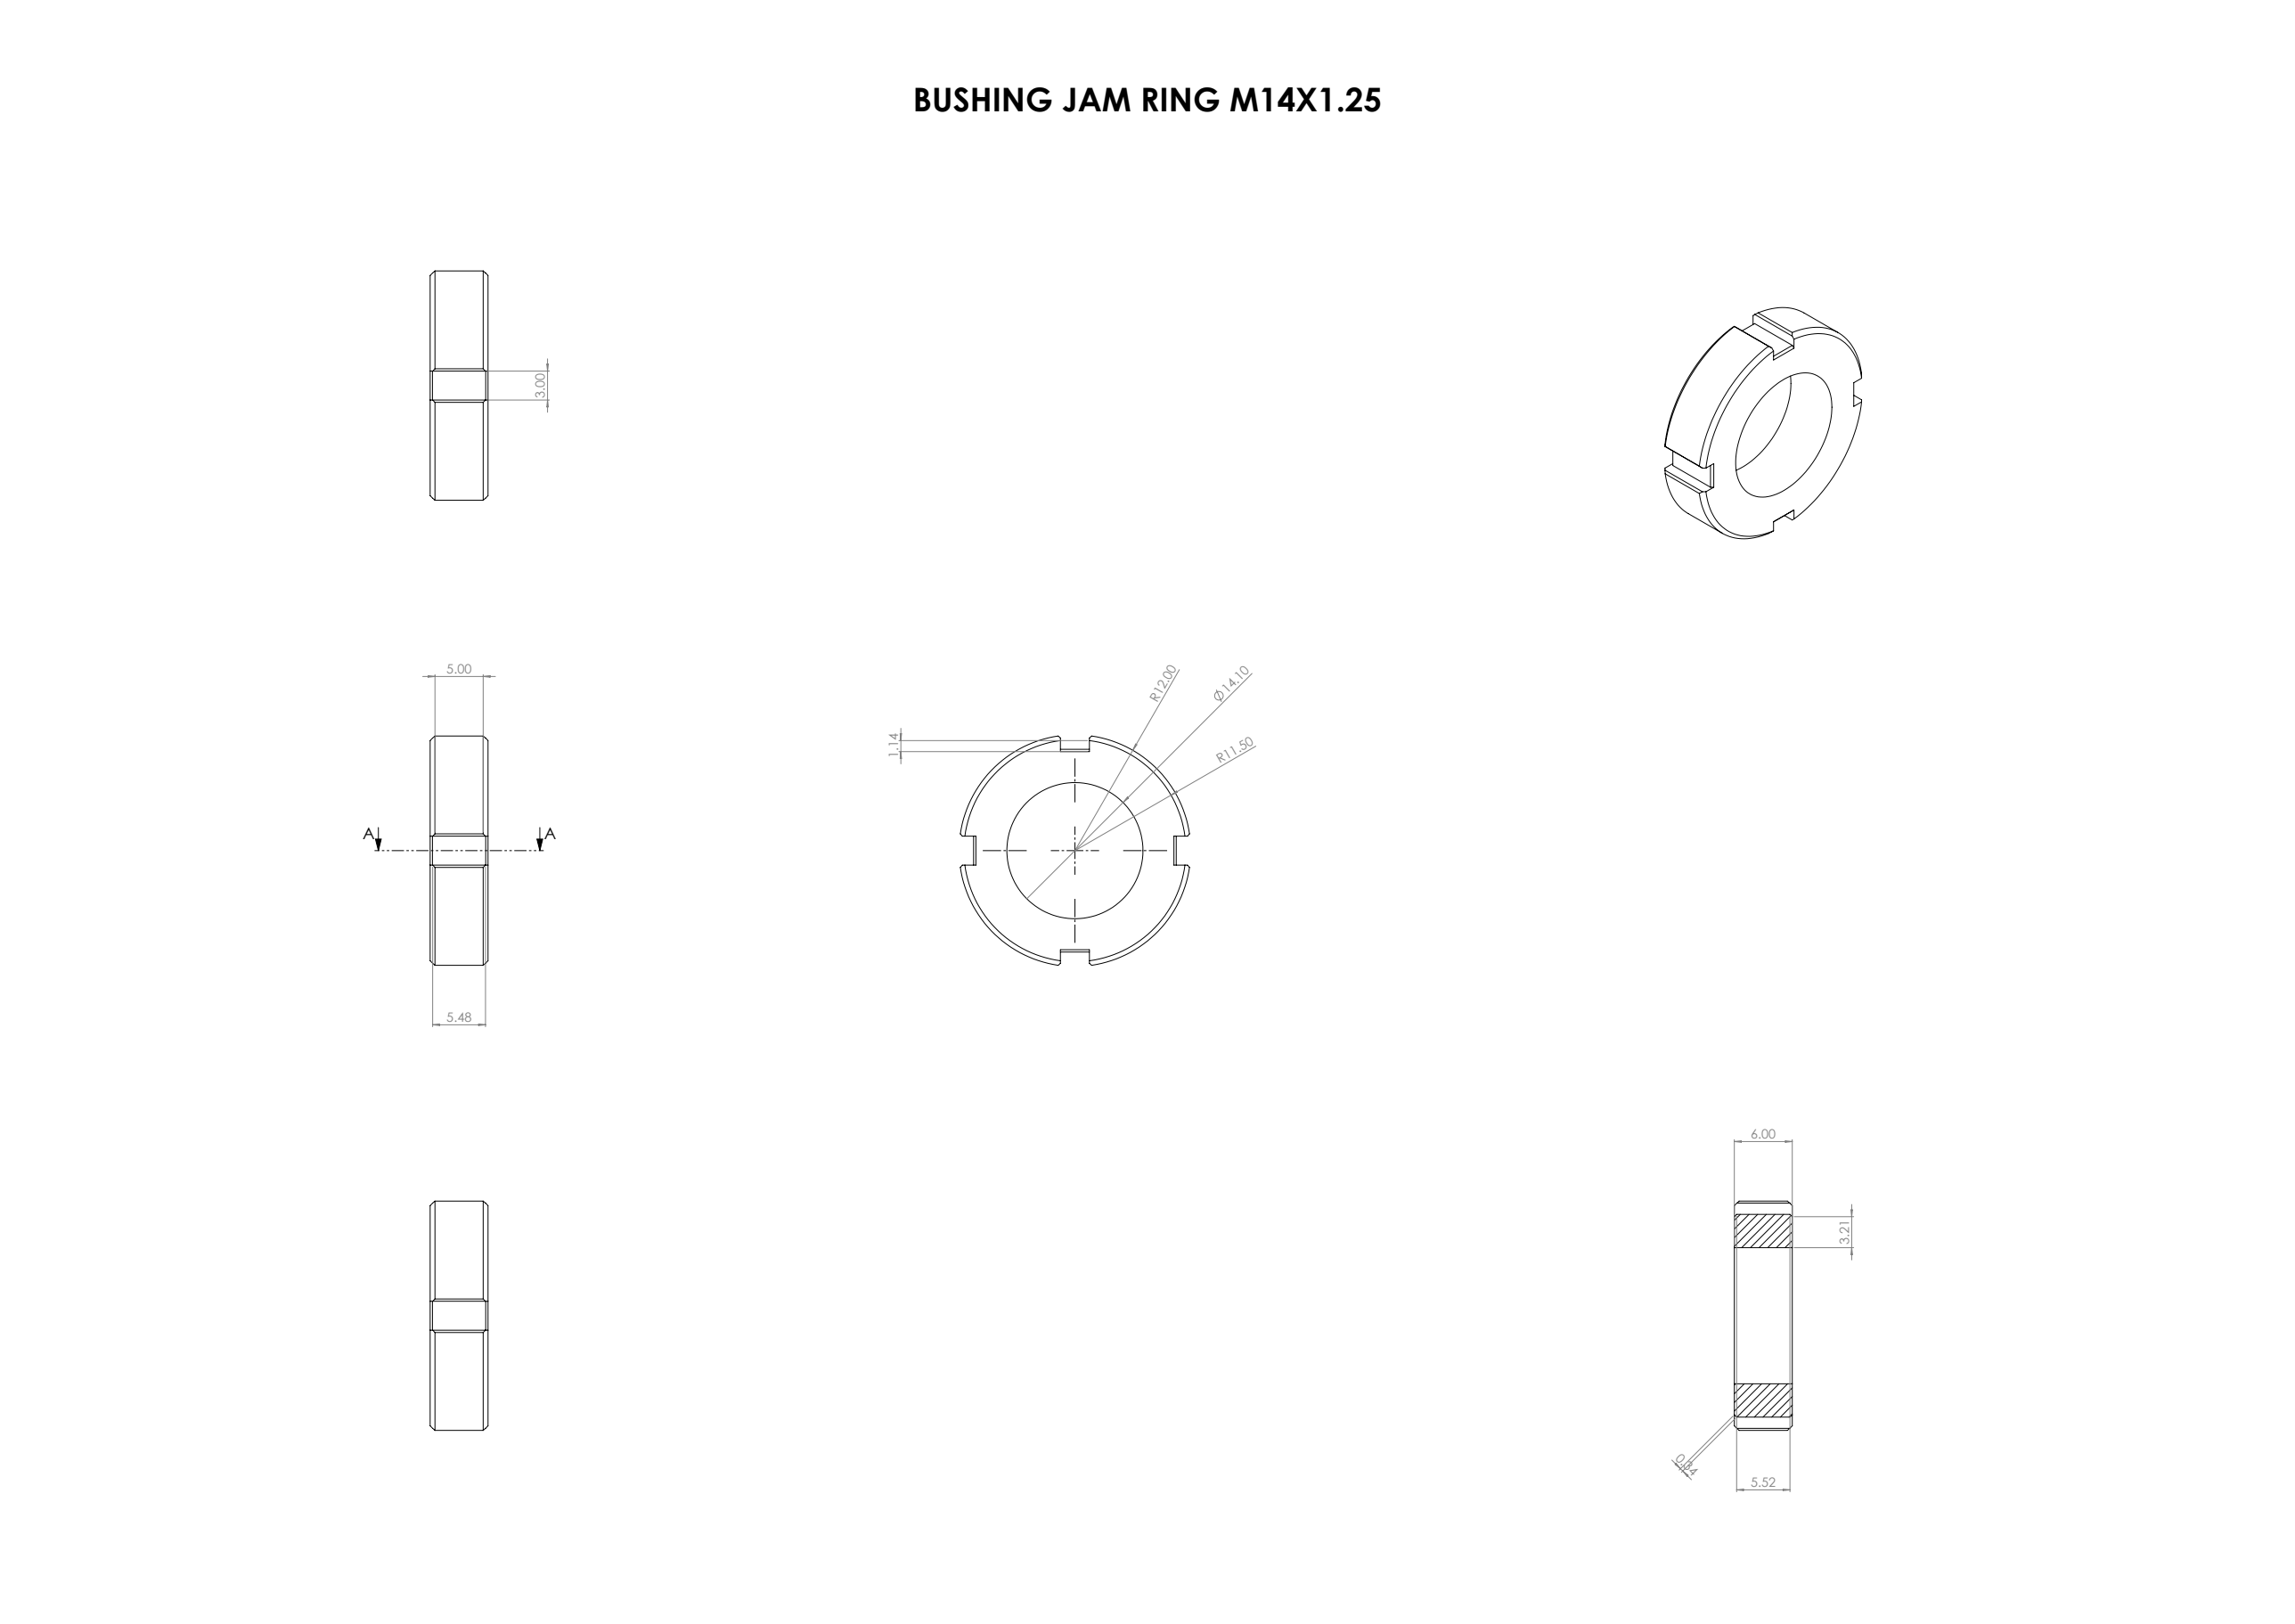
ISO-10303-21;
HEADER;
/* Generated by software containing ST-Developer
 * from STEP Tools, Inc. (www.steptools.com) 
 */

FILE_DESCRIPTION(
/* description */ (''),
/* implementation_level */ '2;1');

FILE_NAME(
/* name */ '08_Bushing_Jam_Ring_M14x1.25.step',
/* time_stamp */ '2026-10-21T01:56:51-07:00',
/* author */ (''),
/* organization */ (''),
/* preprocessor_version */ 'ST-DEVELOPER v20.2',
/* originating_system */ 'Autodesk Translation Framework v15.15.0.0',
/* authorisation */ '');

FILE_SCHEMA (('AUTOMOTIVE_DESIGN { 1 0 10303 214 3 1 1 }'));
ENDSEC;

DATA;
#10=MECHANICAL_DESIGN_GEOMETRIC_PRESENTATION_REPRESENTATION('',(#284),#82384);
#170=(
BOUNDED_CURVE()
B_SPLINE_CURVE(2,(#65757,#65758,#65759),.UNSPECIFIED.,.F.,.F.)
B_SPLINE_CURVE_WITH_KNOTS((3,3),(0.0445378083500862,0.0835095062261198),
 .UNSPECIFIED.)
CURVE()
GEOMETRIC_REPRESENTATION_ITEM()
RATIONAL_B_SPLINE_CURVE((1.00020174547405,1.00018913890855,1.))
REPRESENTATION_ITEM('')
);
#171=(
BOUNDED_CURVE()
B_SPLINE_CURVE(2,(#65763,#65764,#65765),.UNSPECIFIED.,.F.,.F.)
B_SPLINE_CURVE_WITH_KNOTS((3,3),(0.,0.0389716978752448),.UNSPECIFIED.)
CURVE()
GEOMETRIC_REPRESENTATION_ITEM()
RATIONAL_B_SPLINE_CURVE((1.,1.0001891389102,1.00020174547581))
REPRESENTATION_ITEM('')
);
#172=(
BOUNDED_CURVE()
B_SPLINE_CURVE(2,(#65775,#65776,#65777),.UNSPECIFIED.,.F.,.F.)
B_SPLINE_CURVE_WITH_KNOTS((3,3),(0.033425828127436,0.0710030761269733),
 .UNSPECIFIED.)
CURVE()
GEOMETRIC_REPRESENTATION_ITEM()
RATIONAL_B_SPLINE_CURVE((1.0001146955549,1.00012181803223,1.))
REPRESENTATION_ITEM('')
);
#173=(
BOUNDED_CURVE()
B_SPLINE_CURVE(2,(#65781,#65782,#65783),.UNSPECIFIED.,.F.,.F.)
B_SPLINE_CURVE_WITH_KNOTS((3,3),(0.,0.0375772479994726),.UNSPECIFIED.)
CURVE()
GEOMETRIC_REPRESENTATION_ITEM()
RATIONAL_B_SPLINE_CURVE((1.,1.00012181795416,1.0001146954814))
REPRESENTATION_ITEM('')
);
#174=(
BOUNDED_CURVE()
B_SPLINE_CURVE(2,(#65784,#65785,#65786),.UNSPECIFIED.,.F.,.F.)
B_SPLINE_CURVE_WITH_KNOTS((3,3),(0.,0.0389716978752398),.UNSPECIFIED.)
CURVE()
GEOMETRIC_REPRESENTATION_ITEM()
RATIONAL_B_SPLINE_CURVE((1.,1.00018913890916,1.0002017454747))
REPRESENTATION_ITEM('')
);
#175=(
BOUNDED_CURVE()
B_SPLINE_CURVE(2,(#65790,#65791,#65792),.UNSPECIFIED.,.F.,.F.)
B_SPLINE_CURVE_WITH_KNOTS((3,3),(0.0445378083500902,0.0835095062261194),
 .UNSPECIFIED.)
CURVE()
GEOMETRIC_REPRESENTATION_ITEM()
RATIONAL_B_SPLINE_CURVE((1.00020174547445,1.00018913890892,1.))
REPRESENTATION_ITEM('')
);
#176=(
BOUNDED_CURVE()
B_SPLINE_CURVE(2,(#65796,#65797,#65798),.UNSPECIFIED.,.F.,.F.)
B_SPLINE_CURVE_WITH_KNOTS((3,3),(0.,0.0389716978752542),.UNSPECIFIED.)
CURVE()
GEOMETRIC_REPRESENTATION_ITEM()
RATIONAL_B_SPLINE_CURVE((1.,1.00018913890855,1.00020174547405))
REPRESENTATION_ITEM('')
);
#177=(
BOUNDED_CURVE()
B_SPLINE_CURVE(2,(#65802,#65803,#65804),.UNSPECIFIED.,.F.,.F.)
B_SPLINE_CURVE_WITH_KNOTS((3,3),(0.,0.0375772479995372),.UNSPECIFIED.)
CURVE()
GEOMETRIC_REPRESENTATION_ITEM()
RATIONAL_B_SPLINE_CURVE((1.,1.00012181803223,1.0001146955549))
REPRESENTATION_ITEM('')
);
#178=(
BOUNDED_CURVE()
B_SPLINE_CURVE(2,(#65810,#65811,#65812),.UNSPECIFIED.,.F.,.F.)
B_SPLINE_CURVE_WITH_KNOTS((3,3),(0.0334258281258571,0.0710030761269732),
 .UNSPECIFIED.)
CURVE()
GEOMETRIC_REPRESENTATION_ITEM()
RATIONAL_B_SPLINE_CURVE((1.00011469550903,1.00012181798351,1.))
REPRESENTATION_ITEM('')
);
#179=(
BOUNDED_CURVE()
B_SPLINE_CURVE(2,(#65817,#65818,#65819),.UNSPECIFIED.,.F.,.F.)
B_SPLINE_CURVE_WITH_KNOTS((3,3),(0.044537808350094,0.0835095062261198),
 .UNSPECIFIED.)
CURVE()
GEOMETRIC_REPRESENTATION_ITEM()
RATIONAL_B_SPLINE_CURVE((1.00020174547469,1.00018913890915,1.))
REPRESENTATION_ITEM('')
);
#180=(
BOUNDED_CURVE()
B_SPLINE_CURVE(2,(#65821,#65822,#65823),.UNSPECIFIED.,.F.,.F.)
B_SPLINE_CURVE_WITH_KNOTS((3,3),(0.0334258281275199,0.0710030761269733),
 .UNSPECIFIED.)
CURVE()
GEOMETRIC_REPRESENTATION_ITEM()
RATIONAL_B_SPLINE_CURVE((1.00011469547359,1.00012181794587,1.))
REPRESENTATION_ITEM('')
);
#181=(
BOUNDED_CURVE()
B_SPLINE_CURVE(2,(#65844,#65845,#65846),.UNSPECIFIED.,.F.,.F.)
B_SPLINE_CURVE_WITH_KNOTS((3,3),(0.,0.0389716978752325),.UNSPECIFIED.)
CURVE()
GEOMETRIC_REPRESENTATION_ITEM()
RATIONAL_B_SPLINE_CURVE((1.,1.00018913890989,1.00020174547548))
REPRESENTATION_ITEM('')
);
#182=(
BOUNDED_CURVE()
B_SPLINE_CURVE(2,(#65850,#65851,#65852),.UNSPECIFIED.,.F.,.F.)
B_SPLINE_CURVE_WITH_KNOTS((3,3),(0.,0.0375772480011104),.UNSPECIFIED.)
CURVE()
GEOMETRIC_REPRESENTATION_ITEM()
RATIONAL_B_SPLINE_CURVE((1.,1.00012181798092,1.00011469550659))
REPRESENTATION_ITEM('')
);
#183=(
BOUNDED_CURVE()
B_SPLINE_CURVE(2,(#65860,#65861,#65862),.UNSPECIFIED.,.F.,.F.)
B_SPLINE_CURVE_WITH_KNOTS((3,3),(0.0445378083500976,0.0835095062261196),
 .UNSPECIFIED.)
CURVE()
GEOMETRIC_REPRESENTATION_ITEM()
RATIONAL_B_SPLINE_CURVE((1.0002017454746,1.00018913890906,1.))
REPRESENTATION_ITEM('')
);
#184=(
BOUNDED_CURVE()
B_SPLINE_CURVE(2,(#65866,#65867,#65868),.UNSPECIFIED.,.F.,.F.)
B_SPLINE_CURVE_WITH_KNOTS((3,3),(0.,0.0389716978752574),.UNSPECIFIED.)
CURVE()
GEOMETRIC_REPRESENTATION_ITEM()
RATIONAL_B_SPLINE_CURVE((1.,1.00018913890786,1.00020174547332))
REPRESENTATION_ITEM('')
);
#185=(
BOUNDED_CURVE()
B_SPLINE_CURVE(2,(#65878,#65879,#65880),.UNSPECIFIED.,.F.,.F.)
B_SPLINE_CURVE_WITH_KNOTS((3,3),(0.0334258281258531,0.0710030761269732),
 .UNSPECIFIED.)
CURVE()
GEOMETRIC_REPRESENTATION_ITEM()
RATIONAL_B_SPLINE_CURVE((1.00011469551065,1.00012181798524,1.))
REPRESENTATION_ITEM('')
);
#186=(
BOUNDED_CURVE()
B_SPLINE_CURVE(2,(#65884,#65885,#65886),.UNSPECIFIED.,.F.,.F.)
B_SPLINE_CURVE_WITH_KNOTS((3,3),(0.,0.0375772480011044),.UNSPECIFIED.)
CURVE()
GEOMETRIC_REPRESENTATION_ITEM()
RATIONAL_B_SPLINE_CURVE((1.,1.00012181797833,1.00011469550415))
REPRESENTATION_ITEM('')
);
#187=(
BOUNDED_CURVE()
B_SPLINE_CURVE(2,(#65887,#65888,#65889),.UNSPECIFIED.,.F.,.F.)
B_SPLINE_CURVE_WITH_KNOTS((3,3),(0.,0.0389716978752387),.UNSPECIFIED.)
CURVE()
GEOMETRIC_REPRESENTATION_ITEM()
RATIONAL_B_SPLINE_CURVE((1.,1.00018913890938,1.00020174547494))
REPRESENTATION_ITEM('')
);
#188=(
BOUNDED_CURVE()
B_SPLINE_CURVE(2,(#65907,#65908,#65909),.UNSPECIFIED.,.F.,.F.)
B_SPLINE_CURVE_WITH_KNOTS((3,3),(0.0445378083500854,0.0835095062261198),
 .UNSPECIFIED.)
CURVE()
GEOMETRIC_REPRESENTATION_ITEM()
RATIONAL_B_SPLINE_CURVE((1.00020174547577,1.00018913891016,1.))
REPRESENTATION_ITEM('')
);
#189=(
BOUNDED_CURVE()
B_SPLINE_CURVE(2,(#65913,#65914,#65915),.UNSPECIFIED.,.F.,.F.)
B_SPLINE_CURVE_WITH_KNOTS((3,3),(0.0334258281275259,0.0710030761269733),
 .UNSPECIFIED.)
CURVE()
GEOMETRIC_REPRESENTATION_ITEM()
RATIONAL_B_SPLINE_CURVE((1.00011469547113,1.00012181794325,1.))
REPRESENTATION_ITEM('')
);
#190=(
BOUNDED_CURVE()
B_SPLINE_CURVE(2,(#65918,#65919,#65920),.UNSPECIFIED.,.F.,.F.)
B_SPLINE_CURVE_WITH_KNOTS((3,3),(0.,0.0375772479994632),.UNSPECIFIED.)
CURVE()
GEOMETRIC_REPRESENTATION_ITEM()
RATIONAL_B_SPLINE_CURVE((1.,1.00012181795023,1.0001146954777))
REPRESENTATION_ITEM('')
);
#191=(
BOUNDED_CURVE()
B_SPLINE_CURVE(2,(#65929,#65930,#65931),.UNSPECIFIED.,.F.,.F.)
B_SPLINE_CURVE_WITH_KNOTS((3,3),(0.044537808350101,0.0835095062261195),
 .UNSPECIFIED.)
CURVE()
GEOMETRIC_REPRESENTATION_ITEM()
RATIONAL_B_SPLINE_CURVE((1.00020174547522,1.00018913890965,1.))
REPRESENTATION_ITEM('')
);
#192=(
BOUNDED_CURVE()
B_SPLINE_CURVE(2,(#65935,#65936,#65937),.UNSPECIFIED.,.F.,.F.)
B_SPLINE_CURVE_WITH_KNOTS((3,3),(0.,0.0389716978752438),.UNSPECIFIED.)
CURVE()
GEOMETRIC_REPRESENTATION_ITEM()
RATIONAL_B_SPLINE_CURVE((1.,1.00018913890923,1.00020174547478))
REPRESENTATION_ITEM('')
);
#193=(
BOUNDED_CURVE()
B_SPLINE_CURVE(2,(#65947,#65948,#65949),.UNSPECIFIED.,.F.,.F.)
B_SPLINE_CURVE_WITH_KNOTS((3,3),(0.0334258281258831,0.0710030761269732),
 .UNSPECIFIED.)
CURVE()
GEOMETRIC_REPRESENTATION_ITEM()
RATIONAL_B_SPLINE_CURVE((1.00011469550092,1.0001218179749,1.))
REPRESENTATION_ITEM('')
);
#194=(
BOUNDED_CURVE()
B_SPLINE_CURVE(2,(#65953,#65954,#65955),.UNSPECIFIED.,.F.,.F.)
B_SPLINE_CURVE_WITH_KNOTS((3,3),(0.,0.0375772480008883),.UNSPECIFIED.)
CURVE()
GEOMETRIC_REPRESENTATION_ITEM()
RATIONAL_B_SPLINE_CURVE((1.,1.0001218179815,1.00011469550713))
REPRESENTATION_ITEM('')
);
#195=(
BOUNDED_CURVE()
B_SPLINE_CURVE(2,(#65956,#65957,#65958),.UNSPECIFIED.,.F.,.F.)
B_SPLINE_CURVE_WITH_KNOTS((3,3),(0.,0.0389716978752413),.UNSPECIFIED.)
CURVE()
GEOMETRIC_REPRESENTATION_ITEM()
RATIONAL_B_SPLINE_CURVE((1.,1.00018913890951,1.00020174547507))
REPRESENTATION_ITEM('')
);
#196=(
BOUNDED_CURVE()
B_SPLINE_CURVE(2,(#65994,#65995,#65996),.UNSPECIFIED.,.F.,.F.)
B_SPLINE_CURVE_WITH_KNOTS((3,3),(0.0445378083501022,0.0835095062261196),
 .UNSPECIFIED.)
CURVE()
GEOMETRIC_REPRESENTATION_ITEM()
RATIONAL_B_SPLINE_CURVE((1.00020174547498,1.00018913890943,1.))
REPRESENTATION_ITEM('')
);
#197=(
BOUNDED_CURVE()
B_SPLINE_CURVE(2,(#66000,#66001,#66002),.UNSPECIFIED.,.F.,.F.)
B_SPLINE_CURVE_WITH_KNOTS((3,3),(0.0334258281258389,0.0710030761269732),
 .UNSPECIFIED.)
CURVE()
GEOMETRIC_REPRESENTATION_ITEM()
RATIONAL_B_SPLINE_CURVE((1.00011469551635,1.00012181799128,1.))
REPRESENTATION_ITEM('')
);
#198=(
BOUNDED_CURVE()
B_SPLINE_CURVE(2,(#66005,#66006,#66007),.UNSPECIFIED.,.F.,.F.)
B_SPLINE_CURVE_WITH_KNOTS((3,3),(0.,0.0375772480011161),.UNSPECIFIED.)
CURVE()
GEOMETRIC_REPRESENTATION_ITEM()
RATIONAL_B_SPLINE_CURVE((1.,1.00012181798351,1.00011469550903))
REPRESENTATION_ITEM('')
);
#199=(
BOUNDED_CURVE()
B_SPLINE_CURVE(2,(#66013,#66014,#66015),.UNSPECIFIED.,.F.,.F.)
B_SPLINE_CURVE_WITH_KNOTS((3,3),(0.0445378083500857,0.0835095062261197),
 .UNSPECIFIED.)
CURVE()
GEOMETRIC_REPRESENTATION_ITEM()
RATIONAL_B_SPLINE_CURVE((1.00020174547356,1.0001891389081,1.))
REPRESENTATION_ITEM('')
);
#200=(
BOUNDED_CURVE()
B_SPLINE_CURVE(2,(#66019,#66020,#66021),.UNSPECIFIED.,.F.,.F.)
B_SPLINE_CURVE_WITH_KNOTS((3,3),(0.03342582812753,0.0710030761269734),
 .UNSPECIFIED.)
CURVE()
GEOMETRIC_REPRESENTATION_ITEM()
RATIONAL_B_SPLINE_CURVE((1.00011469546948,1.0001218179415,1.))
REPRESENTATION_ITEM('')
);
#201=(
BOUNDED_CURVE()
B_SPLINE_CURVE(2,(#66024,#66025,#66026),.UNSPECIFIED.,.F.,.F.)
B_SPLINE_CURVE_WITH_KNOTS((3,3),(0.,0.0375772479994669),.UNSPECIFIED.)
CURVE()
GEOMETRIC_REPRESENTATION_ITEM()
RATIONAL_B_SPLINE_CURVE((1.,1.00012181795155,1.00011469547894))
REPRESENTATION_ITEM('')
);
#246=SHAPE_REPRESENTATION_RELATIONSHIP('SRR','None',#82480,#265);
#265=ADVANCED_BREP_SHAPE_REPRESENTATION('',(#303),#82379);
#284=STYLED_ITEM('',(#82645),#303);
#303=MANIFOLD_SOLID_BREP('Body1',#30675);
#807=CYLINDRICAL_SURFACE('',#32849,12.);
#808=CYLINDRICAL_SURFACE('',#32864,12.);
#809=CYLINDRICAL_SURFACE('',#32876,12.);
#810=CYLINDRICAL_SURFACE('',#32900,12.);
#811=CYLINDRICAL_SURFACE('',#32904,7.05);
#1724=CIRCLE('',#32850,12.);
#1725=CIRCLE('',#32851,12.);
#1726=CIRCLE('',#32853,11.5);
#1727=CIRCLE('',#32857,12.);
#1728=CIRCLE('',#32858,11.5);
#1729=CIRCLE('',#32865,12.);
#1730=CIRCLE('',#32866,12.);
#1731=CIRCLE('',#32868,11.5);
#1732=CIRCLE('',#32873,11.5);
#1733=CIRCLE('',#32877,12.);
#1734=CIRCLE('',#32878,12.);
#1735=CIRCLE('',#32880,11.5);
#1736=CIRCLE('',#32889,11.5);
#1737=CIRCLE('',#32893,11.5);
#1738=CIRCLE('',#32896,11.5);
#1739=CIRCLE('',#32897,7.05);
#1740=CIRCLE('',#32901,12.);
#1741=CIRCLE('',#32905,7.05);
#2047=CONICAL_SURFACE('',#32852,11.75,0.78539816339745);
#2048=CONICAL_SURFACE('',#32856,11.75,0.78539816339745);
#2049=CONICAL_SURFACE('',#32867,11.75,0.785398163397449);
#2050=CONICAL_SURFACE('',#32872,11.75,0.78539816339745);
#2051=CONICAL_SURFACE('',#32879,11.75,0.785398163397449);
#2052=CONICAL_SURFACE('',#32888,11.75,0.785398163397449);
#2053=CONICAL_SURFACE('',#32892,11.75,0.78539816339745);
#2054=CONICAL_SURFACE('',#32902,11.75,0.785398163397449);
#3564=FACE_BOUND('',#7019,.T.);
#3565=FACE_BOUND('',#7027,.T.);
#4947=FACE_OUTER_BOUND('',#6983,.T.);
#4948=FACE_OUTER_BOUND('',#6984,.T.);
#4949=FACE_OUTER_BOUND('',#6985,.T.);
#4950=FACE_OUTER_BOUND('',#6986,.T.);
#4951=FACE_OUTER_BOUND('',#6987,.T.);
#4952=FACE_OUTER_BOUND('',#6988,.T.);
#4953=FACE_OUTER_BOUND('',#6989,.T.);
#4954=FACE_OUTER_BOUND('',#6990,.T.);
#4955=FACE_OUTER_BOUND('',#6991,.T.);
#4956=FACE_OUTER_BOUND('',#6992,.T.);
#4957=FACE_OUTER_BOUND('',#6993,.T.);
#4958=FACE_OUTER_BOUND('',#6994,.T.);
#4959=FACE_OUTER_BOUND('',#6995,.T.);
#4960=FACE_OUTER_BOUND('',#6996,.T.);
#4961=FACE_OUTER_BOUND('',#6997,.T.);
#4962=FACE_OUTER_BOUND('',#6998,.T.);
#4963=FACE_OUTER_BOUND('',#6999,.T.);
#4964=FACE_OUTER_BOUND('',#7000,.T.);
#4965=FACE_OUTER_BOUND('',#7001,.T.);
#4966=FACE_OUTER_BOUND('',#7002,.T.);
#4967=FACE_OUTER_BOUND('',#7003,.T.);
#4968=FACE_OUTER_BOUND('',#7004,.T.);
#4969=FACE_OUTER_BOUND('',#7005,.T.);
#4970=FACE_OUTER_BOUND('',#7006,.T.);
#4971=FACE_OUTER_BOUND('',#7007,.T.);
#4972=FACE_OUTER_BOUND('',#7008,.T.);
#4973=FACE_OUTER_BOUND('',#7009,.T.);
#4974=FACE_OUTER_BOUND('',#7010,.T.);
#4975=FACE_OUTER_BOUND('',#7011,.T.);
#4976=FACE_OUTER_BOUND('',#7012,.T.);
#4977=FACE_OUTER_BOUND('',#7013,.T.);
#4978=FACE_OUTER_BOUND('',#7014,.T.);
#4979=FACE_OUTER_BOUND('',#7015,.T.);
#4980=FACE_OUTER_BOUND('',#7016,.T.);
#4981=FACE_OUTER_BOUND('',#7017,.T.);
#4982=FACE_OUTER_BOUND('',#7018,.T.);
#4983=FACE_OUTER_BOUND('',#7020,.T.);
#4984=FACE_OUTER_BOUND('',#7021,.T.);
#4985=FACE_OUTER_BOUND('',#7022,.T.);
#4986=FACE_OUTER_BOUND('',#7023,.T.);
#4987=FACE_OUTER_BOUND('',#7024,.T.);
#4988=FACE_OUTER_BOUND('',#7025,.T.);
#4989=FACE_OUTER_BOUND('',#7026,.T.);
#6983=EDGE_LOOP('',(#25917,#25918,#25919,#25920));
#6984=EDGE_LOOP('',(#25921,#25922,#25923,#25924));
#6985=EDGE_LOOP('',(#25925,#25926,#25927,#25928));
#6986=EDGE_LOOP('',(#25929,#25930,#25931,#25932));
#6987=EDGE_LOOP('',(#25933,#25934,#25935,#25936,#25937,#25938));
#6988=EDGE_LOOP('',(#25939,#25940,#25941,#25942));
#6989=EDGE_LOOP('',(#25943,#25944,#25945,#25946,#25947,#25948,#25949,#25950));
#6990=EDGE_LOOP('',(#25951,#25952,#25953,#25954,#25955,#25956));
#6991=EDGE_LOOP('',(#25957,#25958,#25959,#25960));
#6992=EDGE_LOOP('',(#25961,#25962,#25963,#25964));
#6993=EDGE_LOOP('',(#25965,#25966,#25967,#25968));
#6994=EDGE_LOOP('',(#25969,#25970,#25971,#25972,#25973,#25974,#25975,#25976));
#6995=EDGE_LOOP('',(#25977,#25978,#25979,#25980));
#6996=EDGE_LOOP('',(#25981,#25982,#25983,#25984));
#6997=EDGE_LOOP('',(#25985,#25986,#25987,#25988,#25989,#25990));
#6998=EDGE_LOOP('',(#25991,#25992,#25993,#25994));
#6999=EDGE_LOOP('',(#25995,#25996,#25997,#25998));
#7000=EDGE_LOOP('',(#25999,#26000,#26001,#26002));
#7001=EDGE_LOOP('',(#26003,#26004,#26005,#26006,#26007,#26008));
#7002=EDGE_LOOP('',(#26009,#26010,#26011,#26012,#26013,#26014,#26015,#26016));
#7003=EDGE_LOOP('',(#26017,#26018,#26019,#26020));
#7004=EDGE_LOOP('',(#26021,#26022,#26023,#26024));
#7005=EDGE_LOOP('',(#26025,#26026,#26027,#26028,#26029,#26030));
#7006=EDGE_LOOP('',(#26031,#26032,#26033,#26034));
#7007=EDGE_LOOP('',(#26035,#26036,#26037,#26038));
#7008=EDGE_LOOP('',(#26039,#26040,#26041,#26042));
#7009=EDGE_LOOP('',(#26043,#26044,#26045,#26046));
#7010=EDGE_LOOP('',(#26047,#26048,#26049,#26050));
#7011=EDGE_LOOP('',(#26051,#26052,#26053,#26054));
#7012=EDGE_LOOP('',(#26055,#26056,#26057,#26058));
#7013=EDGE_LOOP('',(#26059,#26060,#26061,#26062,#26063,#26064));
#7014=EDGE_LOOP('',(#26065,#26066,#26067,#26068,#26069,#26070,#26071,#26072));
#7015=EDGE_LOOP('',(#26073,#26074,#26075,#26076));
#7016=EDGE_LOOP('',(#26077,#26078,#26079,#26080,#26081,#26082));
#7017=EDGE_LOOP('',(#26083,#26084,#26085,#26086,#26087,#26088,#26089,#26090));
#7018=EDGE_LOOP('',(#26091,#26092,#26093,#26094,#26095,#26096,#26097,#26098,
#26099,#26100,#26101,#26102,#26103,#26104,#26105,#26106));
#7019=EDGE_LOOP('',(#26107));
#7020=EDGE_LOOP('',(#26108,#26109,#26110,#26111,#26112,#26113,#26114,#26115));
#7021=EDGE_LOOP('',(#26116,#26117,#26118,#26119,#26120,#26121,#26122,#26123));
#7022=EDGE_LOOP('',(#26124,#26125,#26126,#26127));
#7023=EDGE_LOOP('',(#26128,#26129,#26130,#26131,#26132,#26133));
#7024=EDGE_LOOP('',(#26134,#26135,#26136,#26137,#26138,#26139,#26140,#26141));
#7025=EDGE_LOOP('',(#26142,#26143,#26144,#26145));
#7026=EDGE_LOOP('',(#26146,#26147,#26148,#26149,#26150,#26151,#26152,#26153,
#26154,#26155,#26156,#26157,#26158,#26159,#26160,#26161));
#7027=EDGE_LOOP('',(#26162));
#9258=LINE('',#65742,#11564);
#9259=LINE('',#65744,#11565);
#9260=LINE('',#65746,#11566);
#9261=LINE('',#65747,#11567);
#9262=LINE('',#65750,#11568);
#9263=LINE('',#65752,#11569);
#9264=LINE('',#65753,#11570);
#9265=LINE('',#65761,#11571);
#9266=LINE('',#65766,#11572);
#9267=LINE('',#65771,#11573);
#9268=LINE('',#65794,#11574);
#9269=LINE('',#65799,#11575);
#9270=LINE('',#65805,#11576);
#9271=LINE('',#65807,#11577);
#9272=LINE('',#65809,#11578);
#9273=LINE('',#65828,#11579);
#9274=LINE('',#65830,#11580);
#9275=LINE('',#65832,#11581);
#9276=LINE('',#65833,#11582);
#9277=LINE('',#65836,#11583);
#9278=LINE('',#65838,#11584);
#9279=LINE('',#65839,#11585);
#9280=LINE('',#65842,#11586);
#9281=LINE('',#65847,#11587);
#9282=LINE('',#65854,#11588);
#9283=LINE('',#65855,#11589);
#9284=LINE('',#65856,#11590);
#9285=LINE('',#65864,#11591);
#9286=LINE('',#65869,#11592);
#9287=LINE('',#65874,#11593);
#9288=LINE('',#65893,#11594);
#9289=LINE('',#65895,#11595);
#9290=LINE('',#65897,#11596);
#9291=LINE('',#65898,#11597);
#9292=LINE('',#65901,#11598);
#9293=LINE('',#65903,#11599);
#9294=LINE('',#65904,#11600);
#9295=LINE('',#65910,#11601);
#9296=LINE('',#65923,#11602);
#9297=LINE('',#65924,#11603);
#9298=LINE('',#65925,#11604);
#9299=LINE('',#65933,#11605);
#9300=LINE('',#65938,#11606);
#9301=LINE('',#65943,#11607);
#9302=LINE('',#65961,#11608);
#9303=LINE('',#65962,#11609);
#9304=LINE('',#65965,#11610);
#9305=LINE('',#65966,#11611);
#9306=LINE('',#65969,#11612);
#9307=LINE('',#65970,#11613);
#9308=LINE('',#65974,#11614);
#9309=LINE('',#65976,#11615);
#9310=LINE('',#65978,#11616);
#9311=LINE('',#65979,#11617);
#9312=LINE('',#65982,#11618);
#9313=LINE('',#65984,#11619);
#9314=LINE('',#65985,#11620);
#9315=LINE('',#65988,#11621);
#9316=LINE('',#65990,#11622);
#9317=LINE('',#65991,#11623);
#9318=LINE('',#65997,#11624);
#9319=LINE('',#66009,#11625);
#9320=LINE('',#66010,#11626);
#9321=LINE('',#66016,#11627);
#9322=LINE('',#66028,#11628);
#9323=LINE('',#66029,#11629);
#9324=LINE('',#66031,#11630);
#9325=LINE('',#66032,#11631);
#9326=LINE('',#66033,#11632);
#9327=LINE('',#66038,#11633);
#9328=LINE('',#66040,#11634);
#9329=LINE('',#66045,#11635);
#9330=LINE('',#66049,#11636);
#11564=VECTOR('',#39203,10.);
#11565=VECTOR('',#39204,10.);
#11566=VECTOR('',#39205,10.);
#11567=VECTOR('',#39206,10.);
#11568=VECTOR('',#39209,10.);
#11569=VECTOR('',#39210,10.);
#11570=VECTOR('',#39211,10.);
#11571=VECTOR('',#39214,10.);
#11572=VECTOR('',#39215,10.);
#11573=VECTOR('',#39220,10.);
#11574=VECTOR('',#39229,10.);
#11575=VECTOR('',#39230,10.);
#11576=VECTOR('',#39233,10.);
#11577=VECTOR('',#39234,10.);
#11578=VECTOR('',#39235,10.);
#11579=VECTOR('',#39244,10.);
#11580=VECTOR('',#39245,10.);
#11581=VECTOR('',#39246,10.);
#11582=VECTOR('',#39247,10.);
#11583=VECTOR('',#39250,10.);
#11584=VECTOR('',#39251,10.);
#11585=VECTOR('',#39252,10.);
#11586=VECTOR('',#39255,10.);
#11587=VECTOR('',#39256,10.);
#11588=VECTOR('',#39259,10.);
#11589=VECTOR('',#39260,10.);
#11590=VECTOR('',#39261,10.);
#11591=VECTOR('',#39264,10.);
#11592=VECTOR('',#39265,10.);
#11593=VECTOR('',#39270,10.);
#11594=VECTOR('',#39279,10.);
#11595=VECTOR('',#39280,10.);
#11596=VECTOR('',#39281,10.);
#11597=VECTOR('',#39282,10.);
#11598=VECTOR('',#39285,10.);
#11599=VECTOR('',#39286,10.);
#11600=VECTOR('',#39287,10.);
#11601=VECTOR('',#39290,10.);
#11602=VECTOR('',#39297,10.);
#11603=VECTOR('',#39298,10.);
#11604=VECTOR('',#39299,10.);
#11605=VECTOR('',#39302,10.);
#11606=VECTOR('',#39303,10.);
#11607=VECTOR('',#39308,10.);
#11608=VECTOR('',#39317,10.);
#11609=VECTOR('',#39318,10.);
#11610=VECTOR('',#39321,10.);
#11611=VECTOR('',#39322,10.);
#11612=VECTOR('',#39325,10.);
#11613=VECTOR('',#39326,10.);
#11614=VECTOR('',#39329,10.);
#11615=VECTOR('',#39330,10.);
#11616=VECTOR('',#39331,10.);
#11617=VECTOR('',#39332,10.);
#11618=VECTOR('',#39335,10.);
#11619=VECTOR('',#39336,10.);
#11620=VECTOR('',#39337,10.);
#11621=VECTOR('',#39340,10.);
#11622=VECTOR('',#39341,10.);
#11623=VECTOR('',#39342,10.);
#11624=VECTOR('',#39345,10.);
#11625=VECTOR('',#39352,10.);
#11626=VECTOR('',#39353,10.);
#11627=VECTOR('',#39356,10.);
#11628=VECTOR('',#39363,10.);
#11629=VECTOR('',#39364,10.);
#11630=VECTOR('',#39367,10.);
#11631=VECTOR('',#39368,10.);
#11632=VECTOR('',#39369,10.);
#11633=VECTOR('',#39376,10.);
#11634=VECTOR('',#39379,10.);
#11635=VECTOR('',#39388,10.);
#11636=VECTOR('',#39393,7.05);
#14136=VERTEX_POINT('',#65740);
#14137=VERTEX_POINT('',#65741);
#14138=VERTEX_POINT('',#65743);
#14139=VERTEX_POINT('',#65745);
#14140=VERTEX_POINT('',#65749);
#14141=VERTEX_POINT('',#65751);
#14142=VERTEX_POINT('',#65755);
#14143=VERTEX_POINT('',#65756);
#14144=VERTEX_POINT('',#65760);
#14145=VERTEX_POINT('',#65762);
#14146=VERTEX_POINT('',#65768);
#14147=VERTEX_POINT('',#65770);
#14148=VERTEX_POINT('',#65774);
#14149=VERTEX_POINT('',#65778);
#14150=VERTEX_POINT('',#65780);
#14151=VERTEX_POINT('',#65788);
#14152=VERTEX_POINT('',#65789);
#14153=VERTEX_POINT('',#65793);
#14154=VERTEX_POINT('',#65795);
#14155=VERTEX_POINT('',#65801);
#14156=VERTEX_POINT('',#65806);
#14157=VERTEX_POINT('',#65808);
#14158=VERTEX_POINT('',#65814);
#14159=VERTEX_POINT('',#65816);
#14160=VERTEX_POINT('',#65820);
#14161=VERTEX_POINT('',#65826);
#14162=VERTEX_POINT('',#65827);
#14163=VERTEX_POINT('',#65829);
#14164=VERTEX_POINT('',#65831);
#14165=VERTEX_POINT('',#65835);
#14166=VERTEX_POINT('',#65837);
#14167=VERTEX_POINT('',#65841);
#14168=VERTEX_POINT('',#65843);
#14169=VERTEX_POINT('',#65849);
#14170=VERTEX_POINT('',#65853);
#14171=VERTEX_POINT('',#65858);
#14172=VERTEX_POINT('',#65859);
#14173=VERTEX_POINT('',#65863);
#14174=VERTEX_POINT('',#65865);
#14175=VERTEX_POINT('',#65871);
#14176=VERTEX_POINT('',#65873);
#14177=VERTEX_POINT('',#65877);
#14178=VERTEX_POINT('',#65881);
#14179=VERTEX_POINT('',#65883);
#14180=VERTEX_POINT('',#65891);
#14181=VERTEX_POINT('',#65892);
#14182=VERTEX_POINT('',#65894);
#14183=VERTEX_POINT('',#65896);
#14184=VERTEX_POINT('',#65900);
#14185=VERTEX_POINT('',#65902);
#14186=VERTEX_POINT('',#65906);
#14187=VERTEX_POINT('',#65912);
#14188=VERTEX_POINT('',#65916);
#14189=VERTEX_POINT('',#65922);
#14190=VERTEX_POINT('',#65927);
#14191=VERTEX_POINT('',#65928);
#14192=VERTEX_POINT('',#65932);
#14193=VERTEX_POINT('',#65934);
#14194=VERTEX_POINT('',#65940);
#14195=VERTEX_POINT('',#65942);
#14196=VERTEX_POINT('',#65946);
#14197=VERTEX_POINT('',#65950);
#14198=VERTEX_POINT('',#65952);
#14199=VERTEX_POINT('',#65960);
#14200=VERTEX_POINT('',#65964);
#14201=VERTEX_POINT('',#65968);
#14202=VERTEX_POINT('',#65972);
#14203=VERTEX_POINT('',#65973);
#14204=VERTEX_POINT('',#65975);
#14205=VERTEX_POINT('',#65977);
#14206=VERTEX_POINT('',#65981);
#14207=VERTEX_POINT('',#65983);
#14208=VERTEX_POINT('',#65987);
#14209=VERTEX_POINT('',#65989);
#14210=VERTEX_POINT('',#65993);
#14211=VERTEX_POINT('',#65999);
#14212=VERTEX_POINT('',#66003);
#14213=VERTEX_POINT('',#66012);
#14214=VERTEX_POINT('',#66018);
#14215=VERTEX_POINT('',#66022);
#14216=VERTEX_POINT('',#66035);
#14217=VERTEX_POINT('',#66047);
#18180=EDGE_CURVE('',#14136,#14137,#9258,.F.);
#18181=EDGE_CURVE('',#14137,#14138,#9259,.T.);
#18182=EDGE_CURVE('',#14138,#14139,#9260,.F.);
#18183=EDGE_CURVE('',#14139,#14136,#9261,.T.);
#18184=EDGE_CURVE('',#14140,#14137,#9262,.T.);
#18185=EDGE_CURVE('',#14141,#14140,#9263,.T.);
#18186=EDGE_CURVE('',#14141,#14138,#9264,.T.);
#18187=EDGE_CURVE('',#14142,#14143,#170,.T.);
#18188=EDGE_CURVE('',#14143,#14144,#9265,.T.);
#18189=EDGE_CURVE('',#14144,#14145,#171,.T.);
#18190=EDGE_CURVE('',#14145,#14142,#9266,.T.);
#18191=EDGE_CURVE('',#14146,#14143,#1724,.T.);
#18192=EDGE_CURVE('',#14147,#14146,#9267,.T.);
#18193=EDGE_CURVE('',#14147,#14144,#1725,.T.);
#18194=EDGE_CURVE('',#14142,#14148,#172,.T.);
#18195=EDGE_CURVE('',#14149,#14148,#1726,.T.);
#18196=EDGE_CURVE('',#14149,#14150,#173,.T.);
#18197=EDGE_CURVE('',#14146,#14150,#174,.T.);
#18198=EDGE_CURVE('',#14151,#14152,#175,.T.);
#18199=EDGE_CURVE('',#14152,#14153,#9268,.T.);
#18200=EDGE_CURVE('',#14153,#14154,#176,.T.);
#18201=EDGE_CURVE('',#14154,#14151,#9269,.T.);
#18202=EDGE_CURVE('',#14155,#14154,#177,.T.);
#18203=EDGE_CURVE('',#14139,#14155,#9270,.T.);
#18204=EDGE_CURVE('',#14156,#14141,#9271,.F.);
#18205=EDGE_CURVE('',#14157,#14156,#9272,.T.);
#18206=EDGE_CURVE('',#14151,#14157,#178,.T.);
#18207=EDGE_CURVE('',#14153,#14158,#1727,.T.);
#18208=EDGE_CURVE('',#14159,#14158,#179,.T.);
#18209=EDGE_CURVE('',#14159,#14160,#180,.T.);
#18210=EDGE_CURVE('',#14155,#14160,#1728,.T.);
#18211=EDGE_CURVE('',#14161,#14162,#9273,.F.);
#18212=EDGE_CURVE('',#14162,#14163,#9274,.T.);
#18213=EDGE_CURVE('',#14163,#14164,#9275,.F.);
#18214=EDGE_CURVE('',#14164,#14161,#9276,.T.);
#18215=EDGE_CURVE('',#14165,#14162,#9277,.T.);
#18216=EDGE_CURVE('',#14166,#14165,#9278,.T.);
#18217=EDGE_CURVE('',#14166,#14163,#9279,.T.);
#18218=EDGE_CURVE('',#14158,#14167,#9280,.T.);
#18219=EDGE_CURVE('',#14167,#14168,#181,.T.);
#18220=EDGE_CURVE('',#14168,#14159,#9281,.T.);
#18221=EDGE_CURVE('',#14169,#14168,#182,.T.);
#18222=EDGE_CURVE('',#14170,#14169,#9282,.T.);
#18223=EDGE_CURVE('',#14165,#14170,#9283,.F.);
#18224=EDGE_CURVE('',#14160,#14161,#9284,.T.);
#18225=EDGE_CURVE('',#14171,#14172,#183,.T.);
#18226=EDGE_CURVE('',#14172,#14173,#9285,.T.);
#18227=EDGE_CURVE('',#14173,#14174,#184,.T.);
#18228=EDGE_CURVE('',#14174,#14171,#9286,.T.);
#18229=EDGE_CURVE('',#14172,#14175,#1729,.T.);
#18230=EDGE_CURVE('',#14176,#14175,#9287,.T.);
#18231=EDGE_CURVE('',#14173,#14176,#1730,.T.);
#18232=EDGE_CURVE('',#14171,#14177,#185,.T.);
#18233=EDGE_CURVE('',#14177,#14178,#1731,.T.);
#18234=EDGE_CURVE('',#14178,#14179,#186,.T.);
#18235=EDGE_CURVE('',#14175,#14179,#187,.T.);
#18236=EDGE_CURVE('',#14180,#14181,#9288,.F.);
#18237=EDGE_CURVE('',#14181,#14182,#9289,.T.);
#18238=EDGE_CURVE('',#14182,#14183,#9290,.F.);
#18239=EDGE_CURVE('',#14183,#14180,#9291,.T.);
#18240=EDGE_CURVE('',#14184,#14181,#9292,.T.);
#18241=EDGE_CURVE('',#14185,#14184,#9293,.T.);
#18242=EDGE_CURVE('',#14185,#14182,#9294,.T.);
#18243=EDGE_CURVE('',#14186,#14176,#188,.T.);
#18244=EDGE_CURVE('',#14179,#14186,#9295,.T.);
#18245=EDGE_CURVE('',#14186,#14187,#189,.T.);
#18246=EDGE_CURVE('',#14188,#14187,#1732,.T.);
#18247=EDGE_CURVE('',#14188,#14174,#190,.T.);
#18248=EDGE_CURVE('',#14189,#14178,#9296,.T.);
#18249=EDGE_CURVE('',#14184,#14189,#9297,.F.);
#18250=EDGE_CURVE('',#14187,#14180,#9298,.T.);
#18251=EDGE_CURVE('',#14190,#14191,#191,.T.);
#18252=EDGE_CURVE('',#14191,#14192,#9299,.T.);
#18253=EDGE_CURVE('',#14192,#14193,#192,.T.);
#18254=EDGE_CURVE('',#14193,#14190,#9300,.T.);
#18255=EDGE_CURVE('',#14191,#14194,#1733,.T.);
#18256=EDGE_CURVE('',#14195,#14194,#9301,.T.);
#18257=EDGE_CURVE('',#14192,#14195,#1734,.T.);
#18258=EDGE_CURVE('',#14190,#14196,#193,.T.);
#18259=EDGE_CURVE('',#14196,#14197,#1735,.T.);
#18260=EDGE_CURVE('',#14197,#14198,#194,.T.);
#18261=EDGE_CURVE('',#14194,#14198,#195,.T.);
#18262=EDGE_CURVE('',#14140,#14199,#9302,.F.);
#18263=EDGE_CURVE('',#14199,#14156,#9303,.T.);
#18264=EDGE_CURVE('',#14200,#14166,#9304,.F.);
#18265=EDGE_CURVE('',#14170,#14200,#9305,.T.);
#18266=EDGE_CURVE('',#14201,#14185,#9306,.F.);
#18267=EDGE_CURVE('',#14189,#14201,#9307,.T.);
#18268=EDGE_CURVE('',#14202,#14203,#9308,.F.);
#18269=EDGE_CURVE('',#14203,#14204,#9309,.T.);
#18270=EDGE_CURVE('',#14204,#14205,#9310,.F.);
#18271=EDGE_CURVE('',#14205,#14202,#9311,.T.);
#18272=EDGE_CURVE('',#14206,#14203,#9312,.T.);
#18273=EDGE_CURVE('',#14207,#14206,#9313,.T.);
#18274=EDGE_CURVE('',#14207,#14204,#9314,.T.);
#18275=EDGE_CURVE('',#14208,#14207,#9315,.F.);
#18276=EDGE_CURVE('',#14206,#14209,#9316,.F.);
#18277=EDGE_CURVE('',#14209,#14208,#9317,.T.);
#18278=EDGE_CURVE('',#14210,#14147,#196,.T.);
#18279=EDGE_CURVE('',#14150,#14210,#9318,.T.);
#18280=EDGE_CURVE('',#14210,#14211,#197,.T.);
#18281=EDGE_CURVE('',#14211,#14212,#1736,.T.);
#18282=EDGE_CURVE('',#14212,#14145,#198,.T.);
#18283=EDGE_CURVE('',#14205,#14149,#9319,.T.);
#18284=EDGE_CURVE('',#14211,#14208,#9320,.T.);
#18285=EDGE_CURVE('',#14213,#14195,#199,.T.);
#18286=EDGE_CURVE('',#14198,#14213,#9321,.T.);
#18287=EDGE_CURVE('',#14213,#14214,#200,.T.);
#18288=EDGE_CURVE('',#14215,#14214,#1737,.T.);
#18289=EDGE_CURVE('',#14215,#14193,#201,.T.);
#18290=EDGE_CURVE('',#14209,#14197,#9322,.T.);
#18291=EDGE_CURVE('',#14214,#14202,#9323,.T.);
#18292=EDGE_CURVE('',#14199,#14212,#9324,.T.);
#18293=EDGE_CURVE('',#14196,#14201,#9325,.T.);
#18294=EDGE_CURVE('',#14177,#14200,#9326,.T.);
#18295=EDGE_CURVE('',#14157,#14169,#1738,.T.);
#18296=EDGE_CURVE('',#14216,#14216,#1739,.T.);
#18297=EDGE_CURVE('',#14183,#14215,#9327,.T.);
#18298=EDGE_CURVE('',#14164,#14188,#9328,.T.);
#18299=EDGE_CURVE('',#14152,#14167,#1740,.T.);
#18300=EDGE_CURVE('',#14148,#14136,#9329,.T.);
#18301=EDGE_CURVE('',#14217,#14217,#1741,.T.);
#18302=EDGE_CURVE('',#14217,#14216,#9330,.T.);
#25917=ORIENTED_EDGE('',*,*,#18180,.T.);
#25918=ORIENTED_EDGE('',*,*,#18181,.T.);
#25919=ORIENTED_EDGE('',*,*,#18182,.T.);
#25920=ORIENTED_EDGE('',*,*,#18183,.T.);
#25921=ORIENTED_EDGE('',*,*,#18181,.F.);
#25922=ORIENTED_EDGE('',*,*,#18184,.F.);
#25923=ORIENTED_EDGE('',*,*,#18185,.F.);
#25924=ORIENTED_EDGE('',*,*,#18186,.T.);
#25925=ORIENTED_EDGE('',*,*,#18187,.T.);
#25926=ORIENTED_EDGE('',*,*,#18188,.T.);
#25927=ORIENTED_EDGE('',*,*,#18189,.T.);
#25928=ORIENTED_EDGE('',*,*,#18190,.T.);
#25929=ORIENTED_EDGE('',*,*,#18188,.F.);
#25930=ORIENTED_EDGE('',*,*,#18191,.F.);
#25931=ORIENTED_EDGE('',*,*,#18192,.F.);
#25932=ORIENTED_EDGE('',*,*,#18193,.T.);
#25933=ORIENTED_EDGE('',*,*,#18187,.F.);
#25934=ORIENTED_EDGE('',*,*,#18194,.T.);
#25935=ORIENTED_EDGE('',*,*,#18195,.F.);
#25936=ORIENTED_EDGE('',*,*,#18196,.T.);
#25937=ORIENTED_EDGE('',*,*,#18197,.F.);
#25938=ORIENTED_EDGE('',*,*,#18191,.T.);
#25939=ORIENTED_EDGE('',*,*,#18198,.T.);
#25940=ORIENTED_EDGE('',*,*,#18199,.T.);
#25941=ORIENTED_EDGE('',*,*,#18200,.T.);
#25942=ORIENTED_EDGE('',*,*,#18201,.T.);
#25943=ORIENTED_EDGE('',*,*,#18201,.F.);
#25944=ORIENTED_EDGE('',*,*,#18202,.F.);
#25945=ORIENTED_EDGE('',*,*,#18203,.F.);
#25946=ORIENTED_EDGE('',*,*,#18182,.F.);
#25947=ORIENTED_EDGE('',*,*,#18186,.F.);
#25948=ORIENTED_EDGE('',*,*,#18204,.F.);
#25949=ORIENTED_EDGE('',*,*,#18205,.F.);
#25950=ORIENTED_EDGE('',*,*,#18206,.F.);
#25951=ORIENTED_EDGE('',*,*,#18200,.F.);
#25952=ORIENTED_EDGE('',*,*,#18207,.T.);
#25953=ORIENTED_EDGE('',*,*,#18208,.F.);
#25954=ORIENTED_EDGE('',*,*,#18209,.T.);
#25955=ORIENTED_EDGE('',*,*,#18210,.F.);
#25956=ORIENTED_EDGE('',*,*,#18202,.T.);
#25957=ORIENTED_EDGE('',*,*,#18211,.T.);
#25958=ORIENTED_EDGE('',*,*,#18212,.T.);
#25959=ORIENTED_EDGE('',*,*,#18213,.T.);
#25960=ORIENTED_EDGE('',*,*,#18214,.T.);
#25961=ORIENTED_EDGE('',*,*,#18212,.F.);
#25962=ORIENTED_EDGE('',*,*,#18215,.F.);
#25963=ORIENTED_EDGE('',*,*,#18216,.F.);
#25964=ORIENTED_EDGE('',*,*,#18217,.T.);
#25965=ORIENTED_EDGE('',*,*,#18208,.T.);
#25966=ORIENTED_EDGE('',*,*,#18218,.T.);
#25967=ORIENTED_EDGE('',*,*,#18219,.T.);
#25968=ORIENTED_EDGE('',*,*,#18220,.T.);
#25969=ORIENTED_EDGE('',*,*,#18220,.F.);
#25970=ORIENTED_EDGE('',*,*,#18221,.F.);
#25971=ORIENTED_EDGE('',*,*,#18222,.F.);
#25972=ORIENTED_EDGE('',*,*,#18223,.F.);
#25973=ORIENTED_EDGE('',*,*,#18215,.T.);
#25974=ORIENTED_EDGE('',*,*,#18211,.F.);
#25975=ORIENTED_EDGE('',*,*,#18224,.F.);
#25976=ORIENTED_EDGE('',*,*,#18209,.F.);
#25977=ORIENTED_EDGE('',*,*,#18225,.T.);
#25978=ORIENTED_EDGE('',*,*,#18226,.T.);
#25979=ORIENTED_EDGE('',*,*,#18227,.T.);
#25980=ORIENTED_EDGE('',*,*,#18228,.T.);
#25981=ORIENTED_EDGE('',*,*,#18226,.F.);
#25982=ORIENTED_EDGE('',*,*,#18229,.T.);
#25983=ORIENTED_EDGE('',*,*,#18230,.F.);
#25984=ORIENTED_EDGE('',*,*,#18231,.F.);
#25985=ORIENTED_EDGE('',*,*,#18225,.F.);
#25986=ORIENTED_EDGE('',*,*,#18232,.T.);
#25987=ORIENTED_EDGE('',*,*,#18233,.T.);
#25988=ORIENTED_EDGE('',*,*,#18234,.T.);
#25989=ORIENTED_EDGE('',*,*,#18235,.F.);
#25990=ORIENTED_EDGE('',*,*,#18229,.F.);
#25991=ORIENTED_EDGE('',*,*,#18236,.T.);
#25992=ORIENTED_EDGE('',*,*,#18237,.T.);
#25993=ORIENTED_EDGE('',*,*,#18238,.T.);
#25994=ORIENTED_EDGE('',*,*,#18239,.T.);
#25995=ORIENTED_EDGE('',*,*,#18237,.F.);
#25996=ORIENTED_EDGE('',*,*,#18240,.F.);
#25997=ORIENTED_EDGE('',*,*,#18241,.F.);
#25998=ORIENTED_EDGE('',*,*,#18242,.T.);
#25999=ORIENTED_EDGE('',*,*,#18243,.T.);
#26000=ORIENTED_EDGE('',*,*,#18230,.T.);
#26001=ORIENTED_EDGE('',*,*,#18235,.T.);
#26002=ORIENTED_EDGE('',*,*,#18244,.T.);
#26003=ORIENTED_EDGE('',*,*,#18227,.F.);
#26004=ORIENTED_EDGE('',*,*,#18231,.T.);
#26005=ORIENTED_EDGE('',*,*,#18243,.F.);
#26006=ORIENTED_EDGE('',*,*,#18245,.T.);
#26007=ORIENTED_EDGE('',*,*,#18246,.F.);
#26008=ORIENTED_EDGE('',*,*,#18247,.T.);
#26009=ORIENTED_EDGE('',*,*,#18244,.F.);
#26010=ORIENTED_EDGE('',*,*,#18234,.F.);
#26011=ORIENTED_EDGE('',*,*,#18248,.F.);
#26012=ORIENTED_EDGE('',*,*,#18249,.F.);
#26013=ORIENTED_EDGE('',*,*,#18240,.T.);
#26014=ORIENTED_EDGE('',*,*,#18236,.F.);
#26015=ORIENTED_EDGE('',*,*,#18250,.F.);
#26016=ORIENTED_EDGE('',*,*,#18245,.F.);
#26017=ORIENTED_EDGE('',*,*,#18251,.T.);
#26018=ORIENTED_EDGE('',*,*,#18252,.T.);
#26019=ORIENTED_EDGE('',*,*,#18253,.T.);
#26020=ORIENTED_EDGE('',*,*,#18254,.T.);
#26021=ORIENTED_EDGE('',*,*,#18252,.F.);
#26022=ORIENTED_EDGE('',*,*,#18255,.T.);
#26023=ORIENTED_EDGE('',*,*,#18256,.F.);
#26024=ORIENTED_EDGE('',*,*,#18257,.F.);
#26025=ORIENTED_EDGE('',*,*,#18251,.F.);
#26026=ORIENTED_EDGE('',*,*,#18258,.T.);
#26027=ORIENTED_EDGE('',*,*,#18259,.T.);
#26028=ORIENTED_EDGE('',*,*,#18260,.T.);
#26029=ORIENTED_EDGE('',*,*,#18261,.F.);
#26030=ORIENTED_EDGE('',*,*,#18255,.F.);
#26031=ORIENTED_EDGE('',*,*,#18204,.T.);
#26032=ORIENTED_EDGE('',*,*,#18185,.T.);
#26033=ORIENTED_EDGE('',*,*,#18262,.T.);
#26034=ORIENTED_EDGE('',*,*,#18263,.T.);
#26035=ORIENTED_EDGE('',*,*,#18264,.T.);
#26036=ORIENTED_EDGE('',*,*,#18216,.T.);
#26037=ORIENTED_EDGE('',*,*,#18223,.T.);
#26038=ORIENTED_EDGE('',*,*,#18265,.T.);
#26039=ORIENTED_EDGE('',*,*,#18266,.T.);
#26040=ORIENTED_EDGE('',*,*,#18241,.T.);
#26041=ORIENTED_EDGE('',*,*,#18249,.T.);
#26042=ORIENTED_EDGE('',*,*,#18267,.T.);
#26043=ORIENTED_EDGE('',*,*,#18268,.T.);
#26044=ORIENTED_EDGE('',*,*,#18269,.T.);
#26045=ORIENTED_EDGE('',*,*,#18270,.T.);
#26046=ORIENTED_EDGE('',*,*,#18271,.T.);
#26047=ORIENTED_EDGE('',*,*,#18269,.F.);
#26048=ORIENTED_EDGE('',*,*,#18272,.F.);
#26049=ORIENTED_EDGE('',*,*,#18273,.F.);
#26050=ORIENTED_EDGE('',*,*,#18274,.T.);
#26051=ORIENTED_EDGE('',*,*,#18275,.T.);
#26052=ORIENTED_EDGE('',*,*,#18273,.T.);
#26053=ORIENTED_EDGE('',*,*,#18276,.T.);
#26054=ORIENTED_EDGE('',*,*,#18277,.T.);
#26055=ORIENTED_EDGE('',*,*,#18278,.T.);
#26056=ORIENTED_EDGE('',*,*,#18192,.T.);
#26057=ORIENTED_EDGE('',*,*,#18197,.T.);
#26058=ORIENTED_EDGE('',*,*,#18279,.T.);
#26059=ORIENTED_EDGE('',*,*,#18189,.F.);
#26060=ORIENTED_EDGE('',*,*,#18193,.F.);
#26061=ORIENTED_EDGE('',*,*,#18278,.F.);
#26062=ORIENTED_EDGE('',*,*,#18280,.T.);
#26063=ORIENTED_EDGE('',*,*,#18281,.T.);
#26064=ORIENTED_EDGE('',*,*,#18282,.T.);
#26065=ORIENTED_EDGE('',*,*,#18279,.F.);
#26066=ORIENTED_EDGE('',*,*,#18196,.F.);
#26067=ORIENTED_EDGE('',*,*,#18283,.F.);
#26068=ORIENTED_EDGE('',*,*,#18270,.F.);
#26069=ORIENTED_EDGE('',*,*,#18274,.F.);
#26070=ORIENTED_EDGE('',*,*,#18275,.F.);
#26071=ORIENTED_EDGE('',*,*,#18284,.F.);
#26072=ORIENTED_EDGE('',*,*,#18280,.F.);
#26073=ORIENTED_EDGE('',*,*,#18285,.T.);
#26074=ORIENTED_EDGE('',*,*,#18256,.T.);
#26075=ORIENTED_EDGE('',*,*,#18261,.T.);
#26076=ORIENTED_EDGE('',*,*,#18286,.T.);
#26077=ORIENTED_EDGE('',*,*,#18253,.F.);
#26078=ORIENTED_EDGE('',*,*,#18257,.T.);
#26079=ORIENTED_EDGE('',*,*,#18285,.F.);
#26080=ORIENTED_EDGE('',*,*,#18287,.T.);
#26081=ORIENTED_EDGE('',*,*,#18288,.F.);
#26082=ORIENTED_EDGE('',*,*,#18289,.T.);
#26083=ORIENTED_EDGE('',*,*,#18286,.F.);
#26084=ORIENTED_EDGE('',*,*,#18260,.F.);
#26085=ORIENTED_EDGE('',*,*,#18290,.F.);
#26086=ORIENTED_EDGE('',*,*,#18276,.F.);
#26087=ORIENTED_EDGE('',*,*,#18272,.T.);
#26088=ORIENTED_EDGE('',*,*,#18268,.F.);
#26089=ORIENTED_EDGE('',*,*,#18291,.F.);
#26090=ORIENTED_EDGE('',*,*,#18287,.F.);
#26091=ORIENTED_EDGE('',*,*,#18292,.T.);
#26092=ORIENTED_EDGE('',*,*,#18281,.F.);
#26093=ORIENTED_EDGE('',*,*,#18284,.T.);
#26094=ORIENTED_EDGE('',*,*,#18277,.F.);
#26095=ORIENTED_EDGE('',*,*,#18290,.T.);
#26096=ORIENTED_EDGE('',*,*,#18259,.F.);
#26097=ORIENTED_EDGE('',*,*,#18293,.T.);
#26098=ORIENTED_EDGE('',*,*,#18267,.F.);
#26099=ORIENTED_EDGE('',*,*,#18248,.T.);
#26100=ORIENTED_EDGE('',*,*,#18233,.F.);
#26101=ORIENTED_EDGE('',*,*,#18294,.T.);
#26102=ORIENTED_EDGE('',*,*,#18265,.F.);
#26103=ORIENTED_EDGE('',*,*,#18222,.T.);
#26104=ORIENTED_EDGE('',*,*,#18295,.F.);
#26105=ORIENTED_EDGE('',*,*,#18205,.T.);
#26106=ORIENTED_EDGE('',*,*,#18263,.F.);
#26107=ORIENTED_EDGE('',*,*,#18296,.T.);
#26108=ORIENTED_EDGE('',*,*,#18254,.F.);
#26109=ORIENTED_EDGE('',*,*,#18289,.F.);
#26110=ORIENTED_EDGE('',*,*,#18297,.F.);
#26111=ORIENTED_EDGE('',*,*,#18238,.F.);
#26112=ORIENTED_EDGE('',*,*,#18242,.F.);
#26113=ORIENTED_EDGE('',*,*,#18266,.F.);
#26114=ORIENTED_EDGE('',*,*,#18293,.F.);
#26115=ORIENTED_EDGE('',*,*,#18258,.F.);
#26116=ORIENTED_EDGE('',*,*,#18228,.F.);
#26117=ORIENTED_EDGE('',*,*,#18247,.F.);
#26118=ORIENTED_EDGE('',*,*,#18298,.F.);
#26119=ORIENTED_EDGE('',*,*,#18213,.F.);
#26120=ORIENTED_EDGE('',*,*,#18217,.F.);
#26121=ORIENTED_EDGE('',*,*,#18264,.F.);
#26122=ORIENTED_EDGE('',*,*,#18294,.F.);
#26123=ORIENTED_EDGE('',*,*,#18232,.F.);
#26124=ORIENTED_EDGE('',*,*,#18199,.F.);
#26125=ORIENTED_EDGE('',*,*,#18299,.T.);
#26126=ORIENTED_EDGE('',*,*,#18218,.F.);
#26127=ORIENTED_EDGE('',*,*,#18207,.F.);
#26128=ORIENTED_EDGE('',*,*,#18198,.F.);
#26129=ORIENTED_EDGE('',*,*,#18206,.T.);
#26130=ORIENTED_EDGE('',*,*,#18295,.T.);
#26131=ORIENTED_EDGE('',*,*,#18221,.T.);
#26132=ORIENTED_EDGE('',*,*,#18219,.F.);
#26133=ORIENTED_EDGE('',*,*,#18299,.F.);
#26134=ORIENTED_EDGE('',*,*,#18190,.F.);
#26135=ORIENTED_EDGE('',*,*,#18282,.F.);
#26136=ORIENTED_EDGE('',*,*,#18292,.F.);
#26137=ORIENTED_EDGE('',*,*,#18262,.F.);
#26138=ORIENTED_EDGE('',*,*,#18184,.T.);
#26139=ORIENTED_EDGE('',*,*,#18180,.F.);
#26140=ORIENTED_EDGE('',*,*,#18300,.F.);
#26141=ORIENTED_EDGE('',*,*,#18194,.F.);
#26142=ORIENTED_EDGE('',*,*,#18301,.T.);
#26143=ORIENTED_EDGE('',*,*,#18302,.T.);
#26144=ORIENTED_EDGE('',*,*,#18296,.F.);
#26145=ORIENTED_EDGE('',*,*,#18302,.F.);
#26146=ORIENTED_EDGE('',*,*,#18203,.T.);
#26147=ORIENTED_EDGE('',*,*,#18210,.T.);
#26148=ORIENTED_EDGE('',*,*,#18224,.T.);
#26149=ORIENTED_EDGE('',*,*,#18214,.F.);
#26150=ORIENTED_EDGE('',*,*,#18298,.T.);
#26151=ORIENTED_EDGE('',*,*,#18246,.T.);
#26152=ORIENTED_EDGE('',*,*,#18250,.T.);
#26153=ORIENTED_EDGE('',*,*,#18239,.F.);
#26154=ORIENTED_EDGE('',*,*,#18297,.T.);
#26155=ORIENTED_EDGE('',*,*,#18288,.T.);
#26156=ORIENTED_EDGE('',*,*,#18291,.T.);
#26157=ORIENTED_EDGE('',*,*,#18271,.F.);
#26158=ORIENTED_EDGE('',*,*,#18283,.T.);
#26159=ORIENTED_EDGE('',*,*,#18195,.T.);
#26160=ORIENTED_EDGE('',*,*,#18300,.T.);
#26161=ORIENTED_EDGE('',*,*,#18183,.F.);
#26162=ORIENTED_EDGE('',*,*,#18301,.F.);
#28792=PLANE('',#32846);
#28793=PLANE('',#32847);
#28794=PLANE('',#32848);
#28795=PLANE('',#32854);
#28796=PLANE('',#32855);
#28797=PLANE('',#32859);
#28798=PLANE('',#32860);
#28799=PLANE('',#32861);
#28800=PLANE('',#32862);
#28801=PLANE('',#32863);
#28802=PLANE('',#32869);
#28803=PLANE('',#32870);
#28804=PLANE('',#32871);
#28805=PLANE('',#32874);
#28806=PLANE('',#32875);
#28807=PLANE('',#32881);
#28808=PLANE('',#32882);
#28809=PLANE('',#32883);
#28810=PLANE('',#32884);
#28811=PLANE('',#32885);
#28812=PLANE('',#32886);
#28813=PLANE('',#32887);
#28814=PLANE('',#32890);
#28815=PLANE('',#32891);
#28816=PLANE('',#32894);
#28817=PLANE('',#32895);
#28818=PLANE('',#32898);
#28819=PLANE('',#32899);
#28820=PLANE('',#32903);
#28821=PLANE('',#32906);
#30275=ADVANCED_FACE('',(#4947),#28792,.T.);
#30276=ADVANCED_FACE('',(#4948),#28793,.F.);
#30277=ADVANCED_FACE('',(#4949),#28794,.T.);
#30278=ADVANCED_FACE('',(#4950),#807,.T.);
#30279=ADVANCED_FACE('',(#4951),#2047,.T.);
#30280=ADVANCED_FACE('',(#4952),#28795,.T.);
#30281=ADVANCED_FACE('',(#4953),#28796,.F.);
#30282=ADVANCED_FACE('',(#4954),#2048,.T.);
#30283=ADVANCED_FACE('',(#4955),#28797,.T.);
#30284=ADVANCED_FACE('',(#4956),#28798,.F.);
#30285=ADVANCED_FACE('',(#4957),#28799,.T.);
#30286=ADVANCED_FACE('',(#4958),#28800,.F.);
#30287=ADVANCED_FACE('',(#4959),#28801,.T.);
#30288=ADVANCED_FACE('',(#4960),#808,.T.);
#30289=ADVANCED_FACE('',(#4961),#2049,.T.);
#30290=ADVANCED_FACE('',(#4962),#28802,.T.);
#30291=ADVANCED_FACE('',(#4963),#28803,.F.);
#30292=ADVANCED_FACE('',(#4964),#28804,.T.);
#30293=ADVANCED_FACE('',(#4965),#2050,.T.);
#30294=ADVANCED_FACE('',(#4966),#28805,.F.);
#30295=ADVANCED_FACE('',(#4967),#28806,.T.);
#30296=ADVANCED_FACE('',(#4968),#809,.T.);
#30297=ADVANCED_FACE('',(#4969),#2051,.T.);
#30298=ADVANCED_FACE('',(#4970),#28807,.T.);
#30299=ADVANCED_FACE('',(#4971),#28808,.T.);
#30300=ADVANCED_FACE('',(#4972),#28809,.T.);
#30301=ADVANCED_FACE('',(#4973),#28810,.T.);
#30302=ADVANCED_FACE('',(#4974),#28811,.F.);
#30303=ADVANCED_FACE('',(#4975),#28812,.T.);
#30304=ADVANCED_FACE('',(#4976),#28813,.T.);
#30305=ADVANCED_FACE('',(#4977),#2052,.T.);
#30306=ADVANCED_FACE('',(#4978),#28814,.F.);
#30307=ADVANCED_FACE('',(#4979),#28815,.T.);
#30308=ADVANCED_FACE('',(#4980),#2053,.T.);
#30309=ADVANCED_FACE('',(#4981),#28816,.F.);
#30310=ADVANCED_FACE('',(#4982,#3564),#28817,.T.);
#30311=ADVANCED_FACE('',(#4983),#28818,.F.);
#30312=ADVANCED_FACE('',(#4984),#28819,.F.);
#30313=ADVANCED_FACE('',(#4985),#810,.T.);
#30314=ADVANCED_FACE('',(#4986),#2054,.T.);
#30315=ADVANCED_FACE('',(#4987),#28820,.F.);
#30316=ADVANCED_FACE('',(#4988),#811,.F.);
#30317=ADVANCED_FACE('',(#4989,#3565),#28821,.T.);
#30675=CLOSED_SHELL('',(#30275,#30276,#30277,#30278,#30279,#30280,#30281,
#30282,#30283,#30284,#30285,#30286,#30287,#30288,#30289,#30290,#30291,#30292,
#30293,#30294,#30295,#30296,#30297,#30298,#30299,#30300,#30301,#30302,#30303,
#30304,#30305,#30306,#30307,#30308,#30309,#30310,#30311,#30312,#30313,#30314,
#30315,#30316,#30317));
#32845=AXIS2_PLACEMENT_3D('',#65738,#39199,#39200);
#32846=AXIS2_PLACEMENT_3D('',#65739,#39201,#39202);
#32847=AXIS2_PLACEMENT_3D('',#65748,#39207,#39208);
#32848=AXIS2_PLACEMENT_3D('',#65754,#39212,#39213);
#32849=AXIS2_PLACEMENT_3D('',#65767,#39216,#39217);
#32850=AXIS2_PLACEMENT_3D('',#65769,#39218,#39219);
#32851=AXIS2_PLACEMENT_3D('',#65772,#39221,#39222);
#32852=AXIS2_PLACEMENT_3D('',#65773,#39223,#39224);
#32853=AXIS2_PLACEMENT_3D('',#65779,#39225,#39226);
#32854=AXIS2_PLACEMENT_3D('',#65787,#39227,#39228);
#32855=AXIS2_PLACEMENT_3D('',#65800,#39231,#39232);
#32856=AXIS2_PLACEMENT_3D('',#65813,#39236,#39237);
#32857=AXIS2_PLACEMENT_3D('',#65815,#39238,#39239);
#32858=AXIS2_PLACEMENT_3D('',#65824,#39240,#39241);
#32859=AXIS2_PLACEMENT_3D('',#65825,#39242,#39243);
#32860=AXIS2_PLACEMENT_3D('',#65834,#39248,#39249);
#32861=AXIS2_PLACEMENT_3D('',#65840,#39253,#39254);
#32862=AXIS2_PLACEMENT_3D('',#65848,#39257,#39258);
#32863=AXIS2_PLACEMENT_3D('',#65857,#39262,#39263);
#32864=AXIS2_PLACEMENT_3D('',#65870,#39266,#39267);
#32865=AXIS2_PLACEMENT_3D('',#65872,#39268,#39269);
#32866=AXIS2_PLACEMENT_3D('',#65875,#39271,#39272);
#32867=AXIS2_PLACEMENT_3D('',#65876,#39273,#39274);
#32868=AXIS2_PLACEMENT_3D('',#65882,#39275,#39276);
#32869=AXIS2_PLACEMENT_3D('',#65890,#39277,#39278);
#32870=AXIS2_PLACEMENT_3D('',#65899,#39283,#39284);
#32871=AXIS2_PLACEMENT_3D('',#65905,#39288,#39289);
#32872=AXIS2_PLACEMENT_3D('',#65911,#39291,#39292);
#32873=AXIS2_PLACEMENT_3D('',#65917,#39293,#39294);
#32874=AXIS2_PLACEMENT_3D('',#65921,#39295,#39296);
#32875=AXIS2_PLACEMENT_3D('',#65926,#39300,#39301);
#32876=AXIS2_PLACEMENT_3D('',#65939,#39304,#39305);
#32877=AXIS2_PLACEMENT_3D('',#65941,#39306,#39307);
#32878=AXIS2_PLACEMENT_3D('',#65944,#39309,#39310);
#32879=AXIS2_PLACEMENT_3D('',#65945,#39311,#39312);
#32880=AXIS2_PLACEMENT_3D('',#65951,#39313,#39314);
#32881=AXIS2_PLACEMENT_3D('',#65959,#39315,#39316);
#32882=AXIS2_PLACEMENT_3D('',#65963,#39319,#39320);
#32883=AXIS2_PLACEMENT_3D('',#65967,#39323,#39324);
#32884=AXIS2_PLACEMENT_3D('',#65971,#39327,#39328);
#32885=AXIS2_PLACEMENT_3D('',#65980,#39333,#39334);
#32886=AXIS2_PLACEMENT_3D('',#65986,#39338,#39339);
#32887=AXIS2_PLACEMENT_3D('',#65992,#39343,#39344);
#32888=AXIS2_PLACEMENT_3D('',#65998,#39346,#39347);
#32889=AXIS2_PLACEMENT_3D('',#66004,#39348,#39349);
#32890=AXIS2_PLACEMENT_3D('',#66008,#39350,#39351);
#32891=AXIS2_PLACEMENT_3D('',#66011,#39354,#39355);
#32892=AXIS2_PLACEMENT_3D('',#66017,#39357,#39358);
#32893=AXIS2_PLACEMENT_3D('',#66023,#39359,#39360);
#32894=AXIS2_PLACEMENT_3D('',#66027,#39361,#39362);
#32895=AXIS2_PLACEMENT_3D('',#66030,#39365,#39366);
#32896=AXIS2_PLACEMENT_3D('',#66034,#39370,#39371);
#32897=AXIS2_PLACEMENT_3D('',#66036,#39372,#39373);
#32898=AXIS2_PLACEMENT_3D('',#66037,#39374,#39375);
#32899=AXIS2_PLACEMENT_3D('',#66039,#39377,#39378);
#32900=AXIS2_PLACEMENT_3D('',#66041,#39380,#39381);
#32901=AXIS2_PLACEMENT_3D('',#66042,#39382,#39383);
#32902=AXIS2_PLACEMENT_3D('',#66043,#39384,#39385);
#32903=AXIS2_PLACEMENT_3D('',#66044,#39386,#39387);
#32904=AXIS2_PLACEMENT_3D('',#66046,#39389,#39390);
#32905=AXIS2_PLACEMENT_3D('',#66048,#39391,#39392);
#32906=AXIS2_PLACEMENT_3D('',#66050,#39394,#39395);
#39199=DIRECTION('axis',(0.,0.,1.));
#39200=DIRECTION('refdir',(1.,0.,0.));
#39201=DIRECTION('center_axis',(0.707106781186548,0.707106781186548,0.));
#39202=DIRECTION('ref_axis',(0.,0.,-1.));
#39203=DIRECTION('',(0.707106781186548,-0.707106781186548,0.));
#39204=DIRECTION('',(0.,0.,1.));
#39205=DIRECTION('',(-0.707106781186548,0.707106781186548,0.));
#39206=DIRECTION('',(0.,0.,-1.));
#39207=DIRECTION('center_axis',(0.,-1.,0.));
#39208=DIRECTION('ref_axis',(0.,0.,-1.));
#39209=DIRECTION('',(1.,0.,0.));
#39210=DIRECTION('',(0.,0.,-1.));
#39211=DIRECTION('',(1.,0.,0.));
#39212=DIRECTION('center_axis',(0.,0.753297855187518,0.657679512657864));
#39213=DIRECTION('ref_axis',(1.,0.,0.));
#39214=DIRECTION('',(-1.,0.,0.));
#39215=DIRECTION('',(1.,0.,0.));
#39216=DIRECTION('center_axis',(1.,0.,0.));
#39217=DIRECTION('ref_axis',(0.,1.,0.));
#39218=DIRECTION('center_axis',(1.,0.,0.));
#39219=DIRECTION('ref_axis',(0.,0.,-1.));
#39220=DIRECTION('',(1.,0.,0.));
#39221=DIRECTION('center_axis',(1.,0.,0.));
#39222=DIRECTION('ref_axis',(0.,0.,-1.));
#39223=DIRECTION('center_axis',(-1.,0.,0.));
#39224=DIRECTION('ref_axis',(0.,1.,0.));
#39225=DIRECTION('center_axis',(1.,0.,0.));
#39226=DIRECTION('ref_axis',(0.,0.,-1.));
#39227=DIRECTION('center_axis',(0.,0.753297855187518,-0.657679512657864));
#39228=DIRECTION('ref_axis',(-1.,0.,0.));
#39229=DIRECTION('',(1.,0.,0.));
#39230=DIRECTION('',(-1.,0.,0.));
#39231=DIRECTION('center_axis',(0.,0.,1.));
#39232=DIRECTION('ref_axis',(0.,-1.,0.));
#39233=DIRECTION('',(0.,1.,0.));
#39234=DIRECTION('',(-0.70710678118655,-0.707106781186545,0.));
#39235=DIRECTION('',(0.,-1.,0.));
#39236=DIRECTION('center_axis',(-1.,0.,0.));
#39237=DIRECTION('ref_axis',(0.,1.,0.));
#39238=DIRECTION('center_axis',(1.,0.,0.));
#39239=DIRECTION('ref_axis',(0.,0.,-1.));
#39240=DIRECTION('center_axis',(1.,0.,0.));
#39241=DIRECTION('ref_axis',(0.,0.,-1.));
#39242=DIRECTION('center_axis',(0.707106781186548,4.32978028117747E-17,
0.707106781186548));
#39243=DIRECTION('ref_axis',(0.707106781186548,0.,-0.707106781186548));
#39244=DIRECTION('',(0.707106781186548,-4.32978028117747E-17,-0.707106781186548));
#39245=DIRECTION('',(0.,-1.,6.12323399573677E-17));
#39246=DIRECTION('',(-0.707106781186548,4.32978028117747E-17,0.707106781186548));
#39247=DIRECTION('',(0.,1.,-6.12323399573677E-17));
#39248=DIRECTION('center_axis',(0.,-6.12323399573677E-17,-1.));
#39249=DIRECTION('ref_axis',(0.,1.,-6.12323399573677E-17));
#39250=DIRECTION('',(1.,0.,0.));
#39251=DIRECTION('',(0.,1.,-6.12323399573677E-17));
#39252=DIRECTION('',(1.,0.,0.));
#39253=DIRECTION('center_axis',(0.,-0.657679512657863,0.753297855187519));
#39254=DIRECTION('ref_axis',(1.,0.,0.));
#39255=DIRECTION('',(-1.,0.,0.));
#39256=DIRECTION('',(1.,0.,0.));
#39257=DIRECTION('center_axis',(0.,1.,-6.12323399573677E-17));
#39258=DIRECTION('ref_axis',(0.,6.12323399573677E-17,1.));
#39259=DIRECTION('',(0.,6.12323399573677E-17,1.));
#39260=DIRECTION('',(0.707106781186547,4.32978028117747E-17,0.707106781186548));
#39261=DIRECTION('',(0.,-6.12323399573677E-17,-1.));
#39262=DIRECTION('center_axis',(0.,0.657679512657864,0.753297855187518));
#39263=DIRECTION('ref_axis',(1.,0.,0.));
#39264=DIRECTION('',(1.,0.,0.));
#39265=DIRECTION('',(-1.,0.,0.));
#39266=DIRECTION('center_axis',(1.,0.,0.));
#39267=DIRECTION('ref_axis',(0.,1.,0.));
#39268=DIRECTION('center_axis',(1.,0.,0.));
#39269=DIRECTION('ref_axis',(0.,0.,-1.));
#39270=DIRECTION('',(-1.,0.,0.));
#39271=DIRECTION('center_axis',(1.,0.,0.));
#39272=DIRECTION('ref_axis',(0.,0.,-1.));
#39273=DIRECTION('center_axis',(1.,0.,0.));
#39274=DIRECTION('ref_axis',(0.,1.,0.));
#39275=DIRECTION('center_axis',(1.,0.,0.));
#39276=DIRECTION('ref_axis',(0.,0.,-1.));
#39277=DIRECTION('center_axis',(0.707106781186548,-0.707106781186548,8.65956056235493E-17));
#39278=DIRECTION('ref_axis',(1.22464679914735E-16,0.,-1.));
#39279=DIRECTION('',(0.707106781186548,0.707106781186548,-8.65956056235493E-17));
#39280=DIRECTION('',(0.,-1.22464679914735E-16,-1.));
#39281=DIRECTION('',(-0.707106781186548,-0.707106781186548,8.65956056235493E-17));
#39282=DIRECTION('',(0.,1.22464679914735E-16,1.));
#39283=DIRECTION('center_axis',(0.,1.,-1.22464679914735E-16));
#39284=DIRECTION('ref_axis',(0.,1.22464679914735E-16,1.));
#39285=DIRECTION('',(1.,0.,0.));
#39286=DIRECTION('',(0.,1.22464679914735E-16,1.));
#39287=DIRECTION('',(1.,0.,0.));
#39288=DIRECTION('center_axis',(0.,-0.753297855187518,-0.657679512657863));
#39289=DIRECTION('ref_axis',(-1.,0.,0.));
#39290=DIRECTION('',(1.,0.,0.));
#39291=DIRECTION('center_axis',(-1.,0.,0.));
#39292=DIRECTION('ref_axis',(0.,1.,0.));
#39293=DIRECTION('center_axis',(1.,0.,0.));
#39294=DIRECTION('ref_axis',(0.,0.,-1.));
#39295=DIRECTION('center_axis',(0.,1.22464679914735E-16,1.));
#39296=DIRECTION('ref_axis',(0.,-1.,1.22464679914735E-16));
#39297=DIRECTION('',(0.,-1.,1.22464679914735E-16));
#39298=DIRECTION('',(0.70710678118655,-0.707106781186545,8.6595605623549E-17));
#39299=DIRECTION('',(0.,1.,-1.22464679914735E-16));
#39300=DIRECTION('center_axis',(0.,-0.753297855187519,0.657679512657863));
#39301=DIRECTION('ref_axis',(1.,0.,0.));
#39302=DIRECTION('',(1.,0.,0.));
#39303=DIRECTION('',(-1.,0.,0.));
#39304=DIRECTION('center_axis',(1.,0.,0.));
#39305=DIRECTION('ref_axis',(0.,1.,0.));
#39306=DIRECTION('center_axis',(1.,0.,0.));
#39307=DIRECTION('ref_axis',(0.,0.,-1.));
#39308=DIRECTION('',(-1.,0.,0.));
#39309=DIRECTION('center_axis',(1.,0.,0.));
#39310=DIRECTION('ref_axis',(0.,0.,-1.));
#39311=DIRECTION('center_axis',(1.,0.,0.));
#39312=DIRECTION('ref_axis',(0.,1.,0.));
#39313=DIRECTION('center_axis',(1.,0.,0.));
#39314=DIRECTION('ref_axis',(0.,0.,-1.));
#39315=DIRECTION('center_axis',(-0.707106781186545,0.70710678118655,0.));
#39316=DIRECTION('ref_axis',(0.,0.,1.));
#39317=DIRECTION('',(0.70710678118655,0.707106781186545,0.));
#39318=DIRECTION('',(0.,0.,1.));
#39319=DIRECTION('center_axis',(-0.707106781186548,4.32978028117746E-17,
0.707106781186547));
#39320=DIRECTION('ref_axis',(0.707106781186547,0.,0.707106781186548));
#39321=DIRECTION('',(-0.707106781186547,-4.32978028117747E-17,-0.707106781186548));
#39322=DIRECTION('',(0.,-1.,6.12323399573677E-17));
#39323=DIRECTION('center_axis',(-0.707106781186545,-0.70710678118655,8.65956056235497E-17));
#39324=DIRECTION('ref_axis',(1.22464679914736E-16,0.,1.));
#39325=DIRECTION('',(-0.70710678118655,0.707106781186545,-8.6595605623549E-17));
#39326=DIRECTION('',(0.,-1.22464679914735E-16,-1.));
#39327=DIRECTION('center_axis',(0.707106781186548,-1.29893408435324E-16,
-0.707106781186548));
#39328=DIRECTION('ref_axis',(-0.707106781186548,0.,-0.707106781186548));
#39329=DIRECTION('',(0.707106781186548,1.29893408435324E-16,0.707106781186548));
#39330=DIRECTION('',(0.,1.,-1.83697019872103E-16));
#39331=DIRECTION('',(-0.707106781186548,-1.29893408435324E-16,-0.707106781186548));
#39332=DIRECTION('',(0.,-1.,1.83697019872103E-16));
#39333=DIRECTION('center_axis',(0.,1.83697019872103E-16,1.));
#39334=DIRECTION('ref_axis',(0.,-1.,1.83697019872103E-16));
#39335=DIRECTION('',(1.,0.,0.));
#39336=DIRECTION('',(0.,-1.,1.83697019872103E-16));
#39337=DIRECTION('',(1.,0.,0.));
#39338=DIRECTION('center_axis',(-0.707106781186545,-1.29893408435325E-16,
-0.70710678118655));
#39339=DIRECTION('ref_axis',(-0.70710678118655,0.,0.707106781186545));
#39340=DIRECTION('',(-0.70710678118655,1.29893408435323E-16,0.707106781186545));
#39341=DIRECTION('',(0.70710678118655,-1.29893408435323E-16,-0.707106781186545));
#39342=DIRECTION('',(0.,1.,-1.83697019872103E-16));
#39343=DIRECTION('center_axis',(0.,-0.657679512657865,-0.753297855187517));
#39344=DIRECTION('ref_axis',(-1.,0.,0.));
#39345=DIRECTION('',(-1.,0.,0.));
#39346=DIRECTION('center_axis',(1.,0.,0.));
#39347=DIRECTION('ref_axis',(0.,1.,0.));
#39348=DIRECTION('center_axis',(1.,0.,0.));
#39349=DIRECTION('ref_axis',(0.,0.,-1.));
#39350=DIRECTION('center_axis',(0.,1.,-1.83697019872103E-16));
#39351=DIRECTION('ref_axis',(0.,1.83697019872103E-16,1.));
#39352=DIRECTION('',(0.,-1.83697019872103E-16,-1.));
#39353=DIRECTION('',(0.,1.83697019872103E-16,1.));
#39354=DIRECTION('center_axis',(0.,0.657679512657864,-0.753297855187518));
#39355=DIRECTION('ref_axis',(-1.,0.,0.));
#39356=DIRECTION('',(1.,0.,0.));
#39357=DIRECTION('center_axis',(-1.,0.,0.));
#39358=DIRECTION('ref_axis',(0.,1.,0.));
#39359=DIRECTION('center_axis',(1.,0.,0.));
#39360=DIRECTION('ref_axis',(0.,0.,-1.));
#39361=DIRECTION('center_axis',(0.,-1.,1.83697019872103E-16));
#39362=DIRECTION('ref_axis',(0.,-1.83697019872103E-16,-1.));
#39363=DIRECTION('',(0.,-1.83697019872103E-16,-1.));
#39364=DIRECTION('',(0.,1.83697019872103E-16,1.));
#39365=DIRECTION('center_axis',(-1.,0.,0.));
#39366=DIRECTION('ref_axis',(0.,0.,1.));
#39367=DIRECTION('',(0.,1.,0.));
#39368=DIRECTION('',(0.,1.,-1.22464679914735E-16));
#39369=DIRECTION('',(0.,-6.12323399573677E-17,-1.));
#39370=DIRECTION('center_axis',(1.,0.,0.));
#39371=DIRECTION('ref_axis',(0.,0.,-1.));
#39372=DIRECTION('center_axis',(1.,0.,0.));
#39373=DIRECTION('ref_axis',(0.,0.,-1.));
#39374=DIRECTION('center_axis',(0.,-1.22464679914735E-16,-1.));
#39375=DIRECTION('ref_axis',(0.,1.,-1.22464679914735E-16));
#39376=DIRECTION('',(0.,-1.,1.22464679914735E-16));
#39377=DIRECTION('center_axis',(0.,-1.,6.12323399573677E-17));
#39378=DIRECTION('ref_axis',(0.,-6.12323399573677E-17,-1.));
#39379=DIRECTION('',(0.,6.12323399573677E-17,1.));
#39380=DIRECTION('center_axis',(1.,0.,0.));
#39381=DIRECTION('ref_axis',(0.,1.,0.));
#39382=DIRECTION('center_axis',(1.,0.,0.));
#39383=DIRECTION('ref_axis',(0.,0.,-1.));
#39384=DIRECTION('center_axis',(1.,0.,0.));
#39385=DIRECTION('ref_axis',(0.,1.,0.));
#39386=DIRECTION('center_axis',(0.,0.,-1.));
#39387=DIRECTION('ref_axis',(0.,1.,0.));
#39388=DIRECTION('',(0.,-1.,0.));
#39389=DIRECTION('center_axis',(1.,0.,0.));
#39390=DIRECTION('ref_axis',(0.,1.,0.));
#39391=DIRECTION('center_axis',(1.,0.,0.));
#39392=DIRECTION('ref_axis',(0.,0.,-1.));
#39393=DIRECTION('',(-1.,0.,0.));
#39394=DIRECTION('center_axis',(1.,0.,0.));
#39395=DIRECTION('ref_axis',(0.,0.,-1.));
#65738=CARTESIAN_POINT('',(0.,0.,0.));
#65739=CARTESIAN_POINT('Origin',(5.88,10.38,0.75));
#65740=CARTESIAN_POINT('',(6.,10.26,-1.5));
#65741=CARTESIAN_POINT('',(5.76,10.5,-1.5));
#65742=CARTESIAN_POINT('',(4.38,11.88,-1.5));
#65743=CARTESIAN_POINT('',(5.76,10.5,1.5));
#65744=CARTESIAN_POINT('',(5.76,10.5,0.75));
#65745=CARTESIAN_POINT('',(6.,10.26,1.5));
#65746=CARTESIAN_POINT('',(3.88,12.38,1.5));
#65747=CARTESIAN_POINT('',(6.,10.26,0.75));
#65748=CARTESIAN_POINT('Origin',(0.,10.5,1.5));
#65749=CARTESIAN_POINT('',(0.24,10.5,-1.5));
#65750=CARTESIAN_POINT('',(0.,10.5,-1.5));
#65751=CARTESIAN_POINT('',(0.24,10.5,1.5));
#65752=CARTESIAN_POINT('',(0.24,10.5,0.75));
#65753=CARTESIAN_POINT('',(0.,10.5,1.5));
#65754=CARTESIAN_POINT('Origin',(3.,11.7696910617194,-1.61890285590863));
#65755=CARTESIAN_POINT('',(5.73807935887593,11.6658808997907,-1.5));
#65756=CARTESIAN_POINT('',(5.5,11.8735012236482,-1.73780571181725));
#65757=CARTESIAN_POINT('Ctrl Pts',(5.73807935887593,11.6658808997907,-1.5));
#65758=CARTESIAN_POINT('Ctrl Pts',(5.62113668491351,11.768650949805,-1.61771152478273));
#65759=CARTESIAN_POINT('Ctrl Pts',(5.5,11.8735012236482,-1.73780571181725));
#65760=CARTESIAN_POINT('',(0.5,11.8735012236482,-1.73780571181725));
#65761=CARTESIAN_POINT('',(3.,11.8735012236482,-1.73780571181725));
#65762=CARTESIAN_POINT('',(0.261920641124074,11.6658808997907,-1.5));
#65763=CARTESIAN_POINT('Ctrl Pts',(0.5,11.8735012236482,-1.73780571181725));
#65764=CARTESIAN_POINT('Ctrl Pts',(0.378863315084015,11.7686509498028,-1.6177115247802));
#65765=CARTESIAN_POINT('Ctrl Pts',(0.261920641124074,11.6658808997907,-1.5));
#65766=CARTESIAN_POINT('',(3.,11.6658808997907,-1.5));
#65767=CARTESIAN_POINT('Origin',(3.,0.,0.));
#65768=CARTESIAN_POINT('',(5.5,1.73780571181725,-11.8735012236482));
#65769=CARTESIAN_POINT('Origin',(5.5,0.,0.));
#65770=CARTESIAN_POINT('',(0.5,1.73780571181725,-11.8735012236482));
#65771=CARTESIAN_POINT('',(3.,1.73780571181725,-11.8735012236482));
#65772=CARTESIAN_POINT('Origin',(0.5,0.,0.));
#65773=CARTESIAN_POINT('Origin',(5.75,0.,0.));
#65774=CARTESIAN_POINT('',(6.,11.4017542509914,-1.5));
#65775=CARTESIAN_POINT('Ctrl Pts',(5.73807935887593,11.6658808997907,-1.5));
#65776=CARTESIAN_POINT('Ctrl Pts',(5.87053918780798,11.5323305910383,-1.5));
#65777=CARTESIAN_POINT('Ctrl Pts',(6.,11.4017542509914,-1.5));
#65778=CARTESIAN_POINT('',(6.,1.5,-11.4017542509914));
#65779=CARTESIAN_POINT('Origin',(6.,0.,0.));
#65780=CARTESIAN_POINT('',(5.73807935887592,1.5,-11.6658808997907));
#65781=CARTESIAN_POINT('Ctrl Pts',(6.,1.5,-11.4017542509914));
#65782=CARTESIAN_POINT('Ctrl Pts',(5.87053918781806,1.5,-11.5323305910281));
#65783=CARTESIAN_POINT('Ctrl Pts',(5.73807935887592,1.5,-11.6658808997907));
#65784=CARTESIAN_POINT('Ctrl Pts',(5.5,1.73780571181725,-11.8735012236482));
#65785=CARTESIAN_POINT('Ctrl Pts',(5.62113668491587,1.61771152478031,-11.7686509498029));
#65786=CARTESIAN_POINT('Ctrl Pts',(5.73807935887592,1.5,-11.6658808997907));
#65787=CARTESIAN_POINT('Origin',(3.,11.7696910617194,1.61890285590863));
#65788=CARTESIAN_POINT('',(0.261920641124074,11.6658808997907,1.5));
#65789=CARTESIAN_POINT('',(0.5,11.8735012236482,1.73780571181725));
#65790=CARTESIAN_POINT('Ctrl Pts',(0.261920641124074,11.6658808997907,1.5));
#65791=CARTESIAN_POINT('Ctrl Pts',(0.378863315086433,11.7686509498049,1.61771152478267));
#65792=CARTESIAN_POINT('Ctrl Pts',(0.5,11.8735012236482,1.73780571181725));
#65793=CARTESIAN_POINT('',(5.5,11.8735012236482,1.73780571181725));
#65794=CARTESIAN_POINT('',(3.,11.8735012236482,1.73780571181725));
#65795=CARTESIAN_POINT('',(5.73807935887593,11.6658808997907,1.5));
#65796=CARTESIAN_POINT('Ctrl Pts',(5.5,11.8735012236482,1.73780571181725));
#65797=CARTESIAN_POINT('Ctrl Pts',(5.62113668491577,11.768650949803,1.61771152478042));
#65798=CARTESIAN_POINT('Ctrl Pts',(5.73807935887593,11.6658808997907,1.5));
#65799=CARTESIAN_POINT('',(3.,11.6658808997907,1.5));
#65800=CARTESIAN_POINT('Origin',(0.,12.5,1.5));
#65801=CARTESIAN_POINT('',(6.,11.4017542509914,1.5));
#65802=CARTESIAN_POINT('Ctrl Pts',(6.,11.4017542509914,1.5));
#65803=CARTESIAN_POINT('Ctrl Pts',(5.87053918780798,11.5323305910383,1.5));
#65804=CARTESIAN_POINT('Ctrl Pts',(5.73807935887593,11.6658808997907,1.5));
#65805=CARTESIAN_POINT('',(6.,9.775,1.5));
#65806=CARTESIAN_POINT('',(0.,10.26,1.5));
#65807=CARTESIAN_POINT('',(0.619999999999999,10.88,1.5));
#65808=CARTESIAN_POINT('',(0.,11.4017542509914,1.5));
#65809=CARTESIAN_POINT('',(0.,12.,1.5));
#65810=CARTESIAN_POINT('Ctrl Pts',(0.261920641124074,11.6658808997907,1.5));
#65811=CARTESIAN_POINT('Ctrl Pts',(0.129460812179182,11.5323305910253,1.5));
#65812=CARTESIAN_POINT('Ctrl Pts',(3.46944695195361E-17,11.4017542509914,
1.5));
#65813=CARTESIAN_POINT('Origin',(5.75,0.,0.));
#65814=CARTESIAN_POINT('',(5.5,1.73780571181725,11.8735012236482));
#65815=CARTESIAN_POINT('Origin',(5.5,0.,0.));
#65816=CARTESIAN_POINT('',(5.73807935887592,1.5,11.6658808997907));
#65817=CARTESIAN_POINT('Ctrl Pts',(5.73807935887592,1.5,11.6658808997907));
#65818=CARTESIAN_POINT('Ctrl Pts',(5.6211366849136,1.61771152478264,11.7686509498049));
#65819=CARTESIAN_POINT('Ctrl Pts',(5.5,1.73780571181725,11.8735012236482));
#65820=CARTESIAN_POINT('',(6.,1.5,11.4017542509914));
#65821=CARTESIAN_POINT('Ctrl Pts',(5.73807935887592,1.5,11.6658808997907));
#65822=CARTESIAN_POINT('Ctrl Pts',(5.87053918781908,1.5,11.5323305910271));
#65823=CARTESIAN_POINT('Ctrl Pts',(6.,1.5,11.4017542509914));
#65824=CARTESIAN_POINT('Origin',(6.,0.,0.));
#65825=CARTESIAN_POINT('Origin',(5.88,2.775,10.38));
#65826=CARTESIAN_POINT('',(6.,1.5,10.26));
#65827=CARTESIAN_POINT('',(5.76,1.5,10.5));
#65828=CARTESIAN_POINT('',(4.38,1.5,11.88));
#65829=CARTESIAN_POINT('',(5.76,-1.5,10.5));
#65830=CARTESIAN_POINT('',(5.76,2.775,10.5));
#65831=CARTESIAN_POINT('',(6.,-1.5,10.26));
#65832=CARTESIAN_POINT('',(3.88,-1.5,12.38));
#65833=CARTESIAN_POINT('',(6.,2.775,10.26));
#65834=CARTESIAN_POINT('Origin',(0.,-1.5,10.5));
#65835=CARTESIAN_POINT('',(0.24,1.5,10.5));
#65836=CARTESIAN_POINT('',(0.,1.5,10.5));
#65837=CARTESIAN_POINT('',(0.24,-1.5,10.5));
#65838=CARTESIAN_POINT('',(0.24,5.,10.5));
#65839=CARTESIAN_POINT('',(0.,-1.5,10.5));
#65840=CARTESIAN_POINT('Origin',(3.,1.61890285590863,11.7696910617194));
#65841=CARTESIAN_POINT('',(0.5,1.73780571181725,11.8735012236482));
#65842=CARTESIAN_POINT('',(3.,1.73780571181725,11.8735012236482));
#65843=CARTESIAN_POINT('',(0.261920641124077,1.5,11.6658808997907));
#65844=CARTESIAN_POINT('Ctrl Pts',(0.500000000000001,1.73780571181725,11.8735012236482));
#65845=CARTESIAN_POINT('Ctrl Pts',(0.378863315084023,1.61771152478021,11.7686509498028));
#65846=CARTESIAN_POINT('Ctrl Pts',(0.261920641124077,1.5,11.6658808997907));
#65847=CARTESIAN_POINT('',(3.,1.5,11.6658808997907));
#65848=CARTESIAN_POINT('Origin',(0.,1.5,10.5));
#65849=CARTESIAN_POINT('',(0.,1.5,11.4017542509914));
#65850=CARTESIAN_POINT('Ctrl Pts',(3.46944695195361E-17,1.5,11.4017542509914));
#65851=CARTESIAN_POINT('Ctrl Pts',(0.129460812178863,1.5,11.532330591025));
#65852=CARTESIAN_POINT('Ctrl Pts',(0.261920641124077,1.5,11.6658808997907));
#65853=CARTESIAN_POINT('',(0.,1.5,10.26));
#65854=CARTESIAN_POINT('',(0.,1.5,5.25));
#65855=CARTESIAN_POINT('',(0.12,1.5,10.38));
#65856=CARTESIAN_POINT('',(6.,1.5,5.25));
#65857=CARTESIAN_POINT('Origin',(3.,-1.61890285590862,11.7696910617194));
#65858=CARTESIAN_POINT('',(0.261920641124075,-1.5,11.6658808997907));
#65859=CARTESIAN_POINT('',(0.5,-1.73780571181725,11.8735012236482));
#65860=CARTESIAN_POINT('Ctrl Pts',(0.261920641124075,-1.5,11.6658808997907));
#65861=CARTESIAN_POINT('Ctrl Pts',(0.378863315086399,-1.61771152478264,
11.7686509498049));
#65862=CARTESIAN_POINT('Ctrl Pts',(0.5,-1.73780571181725,11.8735012236482));
#65863=CARTESIAN_POINT('',(5.5,-1.73780571181725,11.8735012236482));
#65864=CARTESIAN_POINT('',(3.,-1.73780571181725,11.8735012236482));
#65865=CARTESIAN_POINT('',(5.73807935887593,-1.5,11.6658808997907));
#65866=CARTESIAN_POINT('Ctrl Pts',(5.5,-1.73780571181725,11.8735012236482));
#65867=CARTESIAN_POINT('Ctrl Pts',(5.62113668491568,-1.61771152478051,11.7686509498031));
#65868=CARTESIAN_POINT('Ctrl Pts',(5.73807935887593,-1.5,11.6658808997907));
#65869=CARTESIAN_POINT('',(3.,-1.5,11.6658808997907));
#65870=CARTESIAN_POINT('Origin',(3.,0.,0.));
#65871=CARTESIAN_POINT('',(0.5,-11.8735012236482,1.73780571181725));
#65872=CARTESIAN_POINT('Origin',(0.5,0.,0.));
#65873=CARTESIAN_POINT('',(5.5,-11.8735012236482,1.73780571181725));
#65874=CARTESIAN_POINT('',(3.,-11.8735012236482,1.73780571181725));
#65875=CARTESIAN_POINT('Origin',(5.5,0.,0.));
#65876=CARTESIAN_POINT('Origin',(0.25,0.,0.));
#65877=CARTESIAN_POINT('',(0.,-1.5,11.4017542509914));
#65878=CARTESIAN_POINT('Ctrl Pts',(0.261920641124075,-1.5,11.6658808997907));
#65879=CARTESIAN_POINT('Ctrl Pts',(0.129460812179394,-1.5,11.5323305910256));
#65880=CARTESIAN_POINT('Ctrl Pts',(3.46944695195361E-17,-1.5,11.4017542509914));
#65881=CARTESIAN_POINT('',(3.46944695195361E-17,-11.4017542509914,1.5));
#65882=CARTESIAN_POINT('Origin',(0.,0.,0.));
#65883=CARTESIAN_POINT('',(0.261920641124076,-11.6658808997907,1.5));
#65884=CARTESIAN_POINT('Ctrl Pts',(3.46944695195361E-17,-11.4017542509914,
1.5));
#65885=CARTESIAN_POINT('Ctrl Pts',(0.129460812178545,-11.5323305910247,
1.5));
#65886=CARTESIAN_POINT('Ctrl Pts',(0.261920641124076,-11.6658808997907,
1.5));
#65887=CARTESIAN_POINT('Ctrl Pts',(0.5,-11.8735012236482,1.73780571181725));
#65888=CARTESIAN_POINT('Ctrl Pts',(0.378863315084097,-11.7686509498029,
1.61771152478029));
#65889=CARTESIAN_POINT('Ctrl Pts',(0.261920641124076,-11.6658808997907,
1.5));
#65890=CARTESIAN_POINT('Origin',(5.88,-10.38,-0.749999999999998));
#65891=CARTESIAN_POINT('',(6.,-10.26,1.5));
#65892=CARTESIAN_POINT('',(5.76,-10.5,1.5));
#65893=CARTESIAN_POINT('',(4.38,-11.88,1.5));
#65894=CARTESIAN_POINT('',(5.76,-10.5,-1.5));
#65895=CARTESIAN_POINT('',(5.76,-10.5,-0.749999999999998));
#65896=CARTESIAN_POINT('',(6.,-10.26,-1.5));
#65897=CARTESIAN_POINT('',(3.88,-12.38,-1.5));
#65898=CARTESIAN_POINT('',(6.,-10.26,-0.749999999999998));
#65899=CARTESIAN_POINT('Origin',(0.,-10.5,-1.5));
#65900=CARTESIAN_POINT('',(0.24,-10.5,1.5));
#65901=CARTESIAN_POINT('',(0.,-10.5,1.5));
#65902=CARTESIAN_POINT('',(0.24,-10.5,-1.5));
#65903=CARTESIAN_POINT('',(0.24,-10.5,-0.749999999999998));
#65904=CARTESIAN_POINT('',(0.,-10.5,-1.5));
#65905=CARTESIAN_POINT('Origin',(3.,-11.7696910617194,1.61890285590863));
#65906=CARTESIAN_POINT('',(5.73807935887592,-11.6658808997907,1.5));
#65907=CARTESIAN_POINT('Ctrl Pts',(5.73807935887592,-11.6658808997907,1.5));
#65908=CARTESIAN_POINT('Ctrl Pts',(5.6211366849137,-11.7686509498048,1.61771152478254));
#65909=CARTESIAN_POINT('Ctrl Pts',(5.5,-11.8735012236482,1.73780571181725));
#65910=CARTESIAN_POINT('',(3.,-11.6658808997907,1.5));
#65911=CARTESIAN_POINT('Origin',(5.75,0.,0.));
#65912=CARTESIAN_POINT('',(6.,-11.4017542509914,1.5));
#65913=CARTESIAN_POINT('Ctrl Pts',(5.73807935887592,-11.6658808997907,1.5));
#65914=CARTESIAN_POINT('Ctrl Pts',(5.8705391878194,-11.5323305910268,1.5));
#65915=CARTESIAN_POINT('Ctrl Pts',(6.,-11.4017542509914,1.5));
#65916=CARTESIAN_POINT('',(6.,-1.5,11.4017542509914));
#65917=CARTESIAN_POINT('Origin',(6.,0.,0.));
#65918=CARTESIAN_POINT('Ctrl Pts',(6.,-1.5,11.4017542509914));
#65919=CARTESIAN_POINT('Ctrl Pts',(5.87053918781854,-1.5,11.5323305910276));
#65920=CARTESIAN_POINT('Ctrl Pts',(5.73807935887593,-1.5,11.6658808997907));
#65921=CARTESIAN_POINT('Origin',(0.,-10.5,1.5));
#65922=CARTESIAN_POINT('',(0.,-10.26,1.5));
#65923=CARTESIAN_POINT('',(0.,0.499999999999999,1.5));
#65924=CARTESIAN_POINT('',(0.119999999999999,-10.38,1.5));
#65925=CARTESIAN_POINT('',(6.,-1.725,1.5));
#65926=CARTESIAN_POINT('Origin',(3.,-11.7696910617194,-1.61890285590862));
#65927=CARTESIAN_POINT('',(0.261920641124079,-11.6658808997907,-1.5));
#65928=CARTESIAN_POINT('',(0.5,-11.8735012236482,-1.73780571181725));
#65929=CARTESIAN_POINT('Ctrl Pts',(0.261920641124079,-11.6658808997907,
-1.5));
#65930=CARTESIAN_POINT('Ctrl Pts',(0.378863315086326,-11.7686509498049,
-1.61771152478256));
#65931=CARTESIAN_POINT('Ctrl Pts',(0.5,-11.8735012236482,-1.73780571181725));
#65932=CARTESIAN_POINT('',(5.5,-11.8735012236482,-1.73780571181725));
#65933=CARTESIAN_POINT('',(3.,-11.8735012236482,-1.73780571181725));
#65934=CARTESIAN_POINT('',(5.73807935887592,-11.6658808997907,-1.5));
#65935=CARTESIAN_POINT('Ctrl Pts',(5.5,-11.8735012236482,-1.73780571181725));
#65936=CARTESIAN_POINT('Ctrl Pts',(5.62113668491587,-11.7686509498029,-1.61771152478031));
#65937=CARTESIAN_POINT('Ctrl Pts',(5.73807935887592,-11.6658808997907,-1.5));
#65938=CARTESIAN_POINT('',(3.,-11.6658808997907,-1.5));
#65939=CARTESIAN_POINT('Origin',(3.,0.,0.));
#65940=CARTESIAN_POINT('',(0.5,-1.73780571181725,-11.8735012236482));
#65941=CARTESIAN_POINT('Origin',(0.5,0.,0.));
#65942=CARTESIAN_POINT('',(5.5,-1.73780571181725,-11.8735012236482));
#65943=CARTESIAN_POINT('',(3.,-1.73780571181725,-11.8735012236482));
#65944=CARTESIAN_POINT('Origin',(5.5,0.,0.));
#65945=CARTESIAN_POINT('Origin',(0.25,0.,0.));
#65946=CARTESIAN_POINT('',(0.,-11.4017542509914,-1.5));
#65947=CARTESIAN_POINT('Ctrl Pts',(0.261920641124079,-11.6658808997907,
-1.5));
#65948=CARTESIAN_POINT('Ctrl Pts',(0.129460812178151,-11.5323305910243,
-1.5));
#65949=CARTESIAN_POINT('Ctrl Pts',(6.93889390390723E-17,-11.4017542509914,
-1.5));
#65950=CARTESIAN_POINT('',(0.,-1.5,-11.4017542509914));
#65951=CARTESIAN_POINT('Origin',(0.,0.,0.));
#65952=CARTESIAN_POINT('',(0.261920641124077,-1.5,-11.6658808997907));
#65953=CARTESIAN_POINT('Ctrl Pts',(-3.46944695195361E-17,-1.5,-11.4017542509914));
#65954=CARTESIAN_POINT('Ctrl Pts',(0.129460812179839,-1.5,-11.532330591026));
#65955=CARTESIAN_POINT('Ctrl Pts',(0.261920641124077,-1.5,-11.6658808997907));
#65956=CARTESIAN_POINT('Ctrl Pts',(0.5,-1.73780571181725,-11.8735012236482));
#65957=CARTESIAN_POINT('Ctrl Pts',(0.378863315084089,-1.61771152478028,
-11.7686509498029));
#65958=CARTESIAN_POINT('Ctrl Pts',(0.261920641124077,-1.5,-11.6658808997907));
#65959=CARTESIAN_POINT('Origin',(0.12,10.38,0.75));
#65960=CARTESIAN_POINT('',(0.,10.26,-1.5));
#65961=CARTESIAN_POINT('',(0.119999999999999,10.38,-1.5));
#65962=CARTESIAN_POINT('',(0.,10.26,0.75));
#65963=CARTESIAN_POINT('Origin',(0.12,5.,10.38));
#65964=CARTESIAN_POINT('',(0.,-1.5,10.26));
#65965=CARTESIAN_POINT('',(0.62,-1.5,10.88));
#65966=CARTESIAN_POINT('',(0.,5.,10.26));
#65967=CARTESIAN_POINT('Origin',(0.12,-10.38,-0.749999999999998));
#65968=CARTESIAN_POINT('',(0.,-10.26,-1.5));
#65969=CARTESIAN_POINT('',(0.619999999999999,-10.88,-1.5));
#65970=CARTESIAN_POINT('',(0.,-10.26,-0.749999999999998));
#65971=CARTESIAN_POINT('Origin',(5.88,4.275,-10.38));
#65972=CARTESIAN_POINT('',(6.,-1.5,-10.26));
#65973=CARTESIAN_POINT('',(5.76,-1.5,-10.5));
#65974=CARTESIAN_POINT('',(4.38,-1.5,-11.88));
#65975=CARTESIAN_POINT('',(5.76,1.5,-10.5));
#65976=CARTESIAN_POINT('',(5.76,4.275,-10.5));
#65977=CARTESIAN_POINT('',(6.,1.5,-10.26));
#65978=CARTESIAN_POINT('',(3.88,1.5,-12.38));
#65979=CARTESIAN_POINT('',(6.,4.275,-10.26));
#65980=CARTESIAN_POINT('Origin',(0.,1.5,-10.5));
#65981=CARTESIAN_POINT('',(0.24,-1.5,-10.5));
#65982=CARTESIAN_POINT('',(0.,-1.5,-10.5));
#65983=CARTESIAN_POINT('',(0.24,1.5,-10.5));
#65984=CARTESIAN_POINT('',(0.24,6.5,-10.5));
#65985=CARTESIAN_POINT('',(0.,1.5,-10.5));
#65986=CARTESIAN_POINT('Origin',(0.12,6.5,-10.38));
#65987=CARTESIAN_POINT('',(0.,1.5,-10.26));
#65988=CARTESIAN_POINT('',(0.619999999999999,1.5,-10.88));
#65989=CARTESIAN_POINT('',(0.,-1.5,-10.26));
#65990=CARTESIAN_POINT('',(0.12,-1.5,-10.38));
#65991=CARTESIAN_POINT('',(0.,6.5,-10.26));
#65992=CARTESIAN_POINT('Origin',(3.,1.61890285590862,-11.7696910617194));
#65993=CARTESIAN_POINT('',(0.261920641124076,1.5,-11.6658808997907));
#65994=CARTESIAN_POINT('Ctrl Pts',(0.261920641124076,1.5,-11.6658808997907));
#65995=CARTESIAN_POINT('Ctrl Pts',(0.378863315086346,1.61771152478258,-11.7686509498049));
#65996=CARTESIAN_POINT('Ctrl Pts',(0.500000000000001,1.73780571181725,-11.8735012236482));
#65997=CARTESIAN_POINT('',(3.,1.5,-11.6658808997907));
#65998=CARTESIAN_POINT('Origin',(0.25,0.,0.));
#65999=CARTESIAN_POINT('',(0.,1.5,-11.4017542509914));
#66000=CARTESIAN_POINT('Ctrl Pts',(0.261920641124076,1.5,-11.6658808997907));
#66001=CARTESIAN_POINT('Ctrl Pts',(0.129460812180139,1.5,-11.5323305910263));
#66002=CARTESIAN_POINT('Ctrl Pts',(3.46944695195361E-17,1.5,-11.4017542509914));
#66003=CARTESIAN_POINT('',(0.,11.4017542509914,-1.5));
#66004=CARTESIAN_POINT('Origin',(0.,0.,0.));
#66005=CARTESIAN_POINT('Ctrl Pts',(3.46944695195361E-17,11.4017542509914,
-1.5));
#66006=CARTESIAN_POINT('Ctrl Pts',(0.129460812179182,11.5323305910253,-1.5));
#66007=CARTESIAN_POINT('Ctrl Pts',(0.261920641124074,11.6658808997907,-1.5));
#66008=CARTESIAN_POINT('Origin',(0.,1.5,-12.5));
#66009=CARTESIAN_POINT('',(6.,1.5,-6.25));
#66010=CARTESIAN_POINT('',(0.,1.5,-6.25));
#66011=CARTESIAN_POINT('Origin',(3.,-1.61890285590863,-11.7696910617194));
#66012=CARTESIAN_POINT('',(5.73807935887592,-1.5,-11.6658808997907));
#66013=CARTESIAN_POINT('Ctrl Pts',(5.73807935887592,-1.5,-11.6658808997907));
#66014=CARTESIAN_POINT('Ctrl Pts',(5.62113668491346,-1.61771152478279,-11.768650949805));
#66015=CARTESIAN_POINT('Ctrl Pts',(5.5,-1.73780571181725,-11.8735012236482));
#66016=CARTESIAN_POINT('',(3.,-1.5,-11.6658808997907));
#66017=CARTESIAN_POINT('Origin',(5.75,0.,0.));
#66018=CARTESIAN_POINT('',(6.,-1.5,-11.4017542509914));
#66019=CARTESIAN_POINT('Ctrl Pts',(5.73807935887592,-1.5,-11.6658808997907));
#66020=CARTESIAN_POINT('Ctrl Pts',(5.87053918781962,-1.5,-11.5323305910266));
#66021=CARTESIAN_POINT('Ctrl Pts',(6.,-1.5,-11.4017542509914));
#66022=CARTESIAN_POINT('',(6.,-11.4017542509914,-1.5));
#66023=CARTESIAN_POINT('Origin',(6.,0.,0.));
#66024=CARTESIAN_POINT('Ctrl Pts',(6.,-11.4017542509914,-1.5));
#66025=CARTESIAN_POINT('Ctrl Pts',(5.87053918781838,-11.5323305910278,-1.5));
#66026=CARTESIAN_POINT('Ctrl Pts',(5.73807935887592,-11.6658808997907,-1.5));
#66027=CARTESIAN_POINT('Origin',(0.,-1.5,-10.5));
#66028=CARTESIAN_POINT('',(0.,-1.5,-5.25));
#66029=CARTESIAN_POINT('',(6.,-1.5,-5.25));
#66030=CARTESIAN_POINT('Origin',(0.,11.5,0.));
#66031=CARTESIAN_POINT('',(0.,11.,-1.5));
#66032=CARTESIAN_POINT('',(0.,-0.500000000000001,-1.5));
#66033=CARTESIAN_POINT('',(0.,-1.5,6.25));
#66034=CARTESIAN_POINT('Origin',(0.,0.,0.));
#66035=CARTESIAN_POINT('',(0.,-7.05,-8.63375993398884E-16));
#66036=CARTESIAN_POINT('Origin',(0.,0.,0.));
#66037=CARTESIAN_POINT('Origin',(0.,-12.5,-1.5));
#66038=CARTESIAN_POINT('',(6.,-2.725,-1.5));
#66039=CARTESIAN_POINT('Origin',(0.,-1.5,12.5));
#66040=CARTESIAN_POINT('',(6.,-1.5,6.25));
#66041=CARTESIAN_POINT('Origin',(3.,0.,0.));
#66042=CARTESIAN_POINT('Origin',(0.5,0.,0.));
#66043=CARTESIAN_POINT('Origin',(0.25,0.,0.));
#66044=CARTESIAN_POINT('Origin',(0.,10.5,-1.5));
#66045=CARTESIAN_POINT('',(6.,8.775,-1.5));
#66046=CARTESIAN_POINT('Origin',(3.,0.,0.));
#66047=CARTESIAN_POINT('',(6.,-7.05,-8.63375993398884E-16));
#66048=CARTESIAN_POINT('Origin',(6.,0.,0.));
#66049=CARTESIAN_POINT('',(3.,-7.05,-8.63375993398884E-16));
#66050=CARTESIAN_POINT('Origin',(6.,7.05,0.));
#82358=UNCERTAINTY_MEASURE_WITH_UNIT(LENGTH_MEASURE(0.01),#82385,
'DISTANCE_ACCURACY_VALUE',
'Maximum model space distance between geometric entities at asserted c
onnectivities');
#82363=UNCERTAINTY_MEASURE_WITH_UNIT(LENGTH_MEASURE(0.01),#82385,
'DISTANCE_ACCURACY_VALUE',
'Maximum model space distance between geometric entities at asserted c
onnectivities');
#82379=(
GEOMETRIC_REPRESENTATION_CONTEXT(3)
GLOBAL_UNCERTAINTY_ASSIGNED_CONTEXT((#82358))
GLOBAL_UNIT_ASSIGNED_CONTEXT((#82385,#82387,#82388))
REPRESENTATION_CONTEXT('','3D')
);
#82384=(
GEOMETRIC_REPRESENTATION_CONTEXT(3)
GLOBAL_UNCERTAINTY_ASSIGNED_CONTEXT((#82363))
GLOBAL_UNIT_ASSIGNED_CONTEXT((#82385,#82387,#82388))
REPRESENTATION_CONTEXT('','3D')
);
#82385=(
LENGTH_UNIT()
NAMED_UNIT(*)
SI_UNIT(.MILLI.,.METRE.)
);
#82387=(
NAMED_UNIT(*)
PLANE_ANGLE_UNIT()
SI_UNIT($,.RADIAN.)
);
#82388=(
NAMED_UNIT(*)
SI_UNIT($,.STERADIAN.)
SOLID_ANGLE_UNIT()
);
#82404=SHAPE_DEFINITION_REPRESENTATION(#82424,#82480);
#82424=PRODUCT_DEFINITION_SHAPE('',$,#82501);
#82480=SHAPE_REPRESENTATION('',(#32845),#82379);
#82485=PRODUCT_DEFINITION_CONTEXT('part definition',#82547,'design');
#82501=PRODUCT_DEFINITION('2026-10-20-12-38-18-701',
'08_Bushing_Jam_Ring_M14x1.25',#82521,#82485);
#82521=PRODUCT_DEFINITION_FORMATION('',$,#82564);
#82547=APPLICATION_CONTEXT(
'Core Data for Automotive Mechanical Design Process');
#82548=PRODUCT_CONTEXT('part definition',#82547,'mechanical');
#82564=PRODUCT('2026-10-20-12-38-18-701','08_Bushing_Jam_Ring_M14x1.25',
$,(#82548));
#82639=COLOUR_RGB('Off White',0.89,0.88,0.83);
#82640=FILL_AREA_STYLE_COLOUR('',#82639);
#82641=FILL_AREA_STYLE('',(#82640));
#82642=SURFACE_STYLE_FILL_AREA(#82641);
#82643=SURFACE_SIDE_STYLE('',(#82642));
#82644=SURFACE_STYLE_USAGE(.BOTH.,#82643);
#82645=PRESENTATION_STYLE_ASSIGNMENT((#82644));
ENDSEC;
END-ISO-10303-21;
